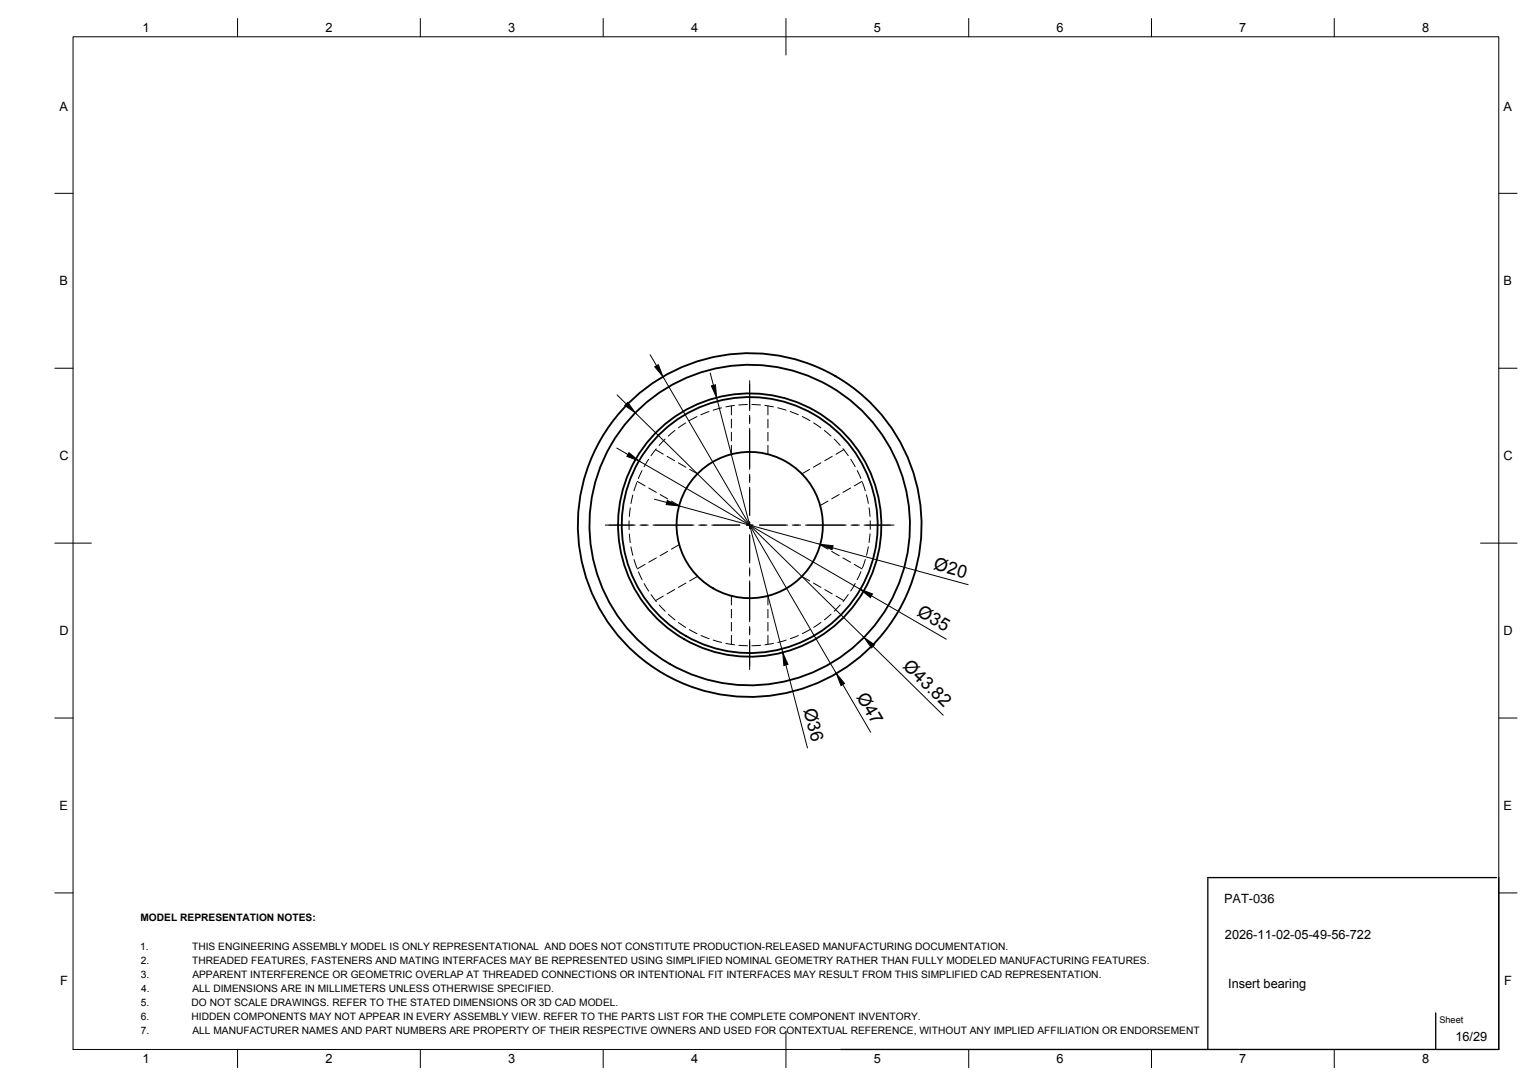
ISO-10303-21;
HEADER;
/* Generated by software containing ST-Developer
 * from STEP Tools, Inc. (www.steptools.com) 
 */

FILE_DESCRIPTION(
/* description */ ('Flange-mounted spindle'),
/* implementation_level */ '2;1');

FILE_NAME(
/* name */ 'Insert bearing.step',
/* time_stamp */ '2026-10-27T10:49:51-07:00',
/* author */ (''),
/* organization */ (''),
/* preprocessor_version */ 'ST-DEVELOPER v20.2',
/* originating_system */ 'Autodesk Translation Framework v15.17.0.0',
/* authorisation */ '');

FILE_SCHEMA (('AUTOMOTIVE_DESIGN { 1 0 10303 214 3 1 1 }'));
ENDSEC;

DATA;
#10=MECHANICAL_DESIGN_GEOMETRIC_PRESENTATION_REPRESENTATION('',(#348,#349),#11764);
#211=B_SPLINE_CURVE_WITH_KNOTS('',3,(#9556,#9557,#9558,#9559,#9560,#9561,
#9562,#9563,#9564,#9565),.UNSPECIFIED.,.F.,.F.,(4,2,2,2,4),(1.13193471301885,
1.22626174930539,1.32058878559194,1.41491753480854,1.50924628402513),
 .UNSPECIFIED.);
#212=B_SPLINE_CURVE_WITH_KNOTS('',3,(#9567,#9568,#9569,#9570,#9571,#9572,
#9573,#9574,#9575,#9576,#9577,#9578,#9579,#9580,#9581,#9582,#9583,#9584),
 .UNSPECIFIED.,.F.,.F.,(4,2,2,2,2,2,2,2,4),(0.377311571006283,0.471638607292829,
0.565965643579376,0.66029439279597,0.754623142012565,0.84895189122916,0.943280640445754,
1.0376076767323,1.13193471301885),.UNSPECIFIED.);
#213=B_SPLINE_CURVE_WITH_KNOTS('',3,(#9585,#9586,#9587,#9588,#9589,#9590,
#9591,#9592,#9593,#9594),.UNSPECIFIED.,.F.,.F.,(4,2,2,2,4),(1.50924628402513,
1.60357503324173,1.69790378245832,1.79223081874487,1.88655785503141),
 .UNSPECIFIED.);
#214=B_SPLINE_CURVE_WITH_KNOTS('',3,(#9597,#9598,#9599,#9600,#9601,#9602,
#9603,#9604,#9605,#9606,#9607,#9608,#9609,#9610,#9611,#9612,#9613,#9614,
#9615,#9616,#9617,#9618,#9619,#9620,#9621,#9622,#9623,#9624,#9625,#9626,
#9627,#9628,#9629,#9630),.UNSPECIFIED.,.T.,.F.,(4,2,2,2,2,2,2,2,2,2,2,2,
2,2,2,2,4),(0.,0.0946120580087934,0.189224116017587,0.283822945575014,0.378421775132442,
0.47302060468987,0.567619434247297,0.662231492256091,0.756843550264884,
0.851455608273677,0.94606766628247,1.0406664958399,1.13526532539733,1.22986415495475,
1.32446298451218,1.41907504252097,1.51368710052977),.UNSPECIFIED.);
#215=B_SPLINE_CURVE_WITH_KNOTS('',3,(#9633,#9634,#9635,#9636,#9637,#9638,
#9639,#9640,#9641,#9642,#9643,#9644,#9645,#9646,#9647,#9648,#9649,#9650,
#9651,#9652,#9653,#9654,#9655,#9656,#9657,#9658,#9659,#9660,#9661,#9662,
#9663,#9664,#9665,#9666),.UNSPECIFIED.,.T.,.F.,(4,2,2,2,2,2,2,2,2,2,2,2,
2,2,2,2,4),(0.,0.0946120580087934,0.189224116017587,0.283822945575014,0.378421775132442,
0.47302060468987,0.567619434247297,0.66223149225609,0.756843550264884,0.851455608273677,
0.94606766628247,1.0406664958399,1.13526532539733,1.22986415495475,1.32446298451218,
1.41907504252097,1.51368710052977),.UNSPECIFIED.);
#216=B_SPLINE_CURVE_WITH_KNOTS('',3,(#9670,#9671,#9672,#9673,#9674,#9675,
#9676,#9677,#9678,#9679),.UNSPECIFIED.,.F.,.F.,(4,2,2,2,4),(1.13193471301885,
1.22626174930539,1.32058878559194,1.41491753480854,1.50924628402513),
 .UNSPECIFIED.);
#217=B_SPLINE_CURVE_WITH_KNOTS('',3,(#9681,#9682,#9683,#9684,#9685,#9686,
#9687,#9688,#9689,#9690,#9691,#9692,#9693,#9694,#9695,#9696,#9697,#9698),
 .UNSPECIFIED.,.F.,.F.,(4,2,2,2,2,2,2,2,4),(0.377311571006283,0.47163860729283,
0.565965643579376,0.660294392795971,0.754623142012565,0.84895189122916,
0.943280640445755,1.0376076767323,1.13193471301885),.UNSPECIFIED.);
#218=B_SPLINE_CURVE_WITH_KNOTS('',3,(#9699,#9700,#9701,#9702,#9703,#9704,
#9705,#9706,#9707,#9708),.UNSPECIFIED.,.F.,.F.,(4,2,2,2,4),(1.50924628402513,
1.60357503324173,1.69790378245832,1.79223081874487,1.88655785503141),
 .UNSPECIFIED.);
#219=B_SPLINE_CURVE_WITH_KNOTS('',3,(#9717,#9718,#9719,#9720,#9721,#9722,
#9723,#9724,#9725,#9726,#9727,#9728,#9729,#9730,#9731,#9732,#9733,#9734),
 .UNSPECIFIED.,.F.,.F.,(4,2,2,2,2,2,2,2,4),(0.377311571006282,0.471638607292829,
0.565965643579376,0.660294392795971,0.754623142012565,0.84895189122916,
0.943280640445754,1.0376076767323,1.13193471301885),.UNSPECIFIED.);
#220=B_SPLINE_CURVE_WITH_KNOTS('',3,(#9736,#9737,#9738,#9739,#9740,#9741,
#9742,#9743,#9744,#9745),.UNSPECIFIED.,.F.,.F.,(4,2,2,2,4),(1.13193471301885,
1.22626174930539,1.32058878559194,1.41491753480854,1.50924628402513),
 .UNSPECIFIED.);
#221=B_SPLINE_CURVE_WITH_KNOTS('',3,(#9746,#9747,#9748,#9749,#9750,#9751,
#9752,#9753,#9754,#9755),.UNSPECIFIED.,.F.,.F.,(4,2,2,2,4),(1.50924628402513,
1.60357503324172,1.69790378245832,1.79223081874487,1.88655785503141),
 .UNSPECIFIED.);
#222=B_SPLINE_CURVE_WITH_KNOTS('',3,(#9758,#9759,#9760,#9761,#9762,#9763,
#9764,#9765,#9766,#9767,#9768,#9769,#9770,#9771,#9772,#9773,#9774,#9775),
 .UNSPECIFIED.,.F.,.F.,(4,2,2,2,2,2,2,2,4),(0.377311571006283,0.47163860729283,
0.565965643579376,0.660294392795971,0.754623142012565,0.84895189122916,
0.943280640445754,1.0376076767323,1.13193471301885),.UNSPECIFIED.);
#223=B_SPLINE_CURVE_WITH_KNOTS('',3,(#9777,#9778,#9779,#9780,#9781,#9782,
#9783,#9784,#9785,#9786),.UNSPECIFIED.,.F.,.F.,(4,2,2,2,4),(1.13193471301885,
1.22626174930539,1.32058878559194,1.41491753480854,1.50924628402513),
 .UNSPECIFIED.);
#224=B_SPLINE_CURVE_WITH_KNOTS('',3,(#9787,#9788,#9789,#9790,#9791,#9792,
#9793,#9794,#9795,#9796),.UNSPECIFIED.,.F.,.F.,(4,2,2,2,4),(1.50924628402513,
1.60357503324173,1.69790378245832,1.79223081874487,1.88655785503141),
 .UNSPECIFIED.);
#225=B_SPLINE_CURVE_WITH_KNOTS('',3,(#9799,#9800,#9801,#9802,#9803,#9804,
#9805,#9806,#9807,#9808,#9809,#9810,#9811,#9812,#9813,#9814,#9815,#9816),
 .UNSPECIFIED.,.F.,.F.,(4,2,2,2,2,2,2,2,4),(0.377311571006282,0.471638607292829,
0.565965643579376,0.66029439279597,0.754623142012565,0.84895189122916,0.943280640445754,
1.0376076767323,1.13193471301885),.UNSPECIFIED.);
#226=B_SPLINE_CURVE_WITH_KNOTS('',3,(#9818,#9819,#9820,#9821,#9822,#9823,
#9824,#9825,#9826,#9827),.UNSPECIFIED.,.F.,.F.,(4,2,2,2,4),(1.13193471301885,
1.22626174930539,1.32058878559194,1.41491753480854,1.50924628402513),
 .UNSPECIFIED.);
#227=B_SPLINE_CURVE_WITH_KNOTS('',3,(#9828,#9829,#9830,#9831,#9832,#9833,
#9834,#9835,#9836,#9837),.UNSPECIFIED.,.F.,.F.,(4,2,2,2,4),(1.50924628402513,
1.60357503324172,1.69790378245832,1.79223081874487,1.88655785503141),
 .UNSPECIFIED.);
#228=B_SPLINE_CURVE_WITH_KNOTS('',3,(#9840,#9841,#9842,#9843,#9844,#9845,
#9846,#9847,#9848,#9849,#9850,#9851,#9852,#9853,#9854,#9855,#9856,#9857),
 .UNSPECIFIED.,.F.,.F.,(4,2,2,2,2,2,2,2,4),(0.377311571006283,0.471638607292829,
0.565965643579376,0.660294392795971,0.754623142012565,0.84895189122916,
0.943280640445755,1.0376076767323,1.13193471301885),.UNSPECIFIED.);
#229=B_SPLINE_CURVE_WITH_KNOTS('',3,(#9859,#9860,#9861,#9862,#9863,#9864,
#9865,#9866,#9867,#9868),.UNSPECIFIED.,.F.,.F.,(4,2,2,2,4),(1.13193471301885,
1.22626174930539,1.32058878559194,1.41491753480854,1.50924628402513),
 .UNSPECIFIED.);
#230=B_SPLINE_CURVE_WITH_KNOTS('',3,(#9869,#9870,#9871,#9872,#9873,#9874,
#9875,#9876,#9877,#9878),.UNSPECIFIED.,.F.,.F.,(4,2,2,2,4),(1.50924628402513,
1.60357503324172,1.69790378245832,1.79223081874487,1.88655785503141),
 .UNSPECIFIED.);
#231=B_SPLINE_CURVE_WITH_KNOTS('',3,(#9882,#9883,#9884,#9885,#9886,#9887,
#9888,#9889,#9890,#9891,#9892,#9893,#9894,#9895,#9896,#9897,#9898,#9899,
#9900,#9901,#9902,#9903,#9904,#9905,#9906,#9907,#9908,#9909,#9910,#9911,
#9912,#9913,#9914,#9915),.UNSPECIFIED.,.T.,.F.,(4,2,2,2,2,2,2,2,2,2,2,2,
2,2,2,2,4),(0.,0.0946120580087934,0.189224116017587,0.283822945575014,0.378421775132442,
0.47302060468987,0.567619434247297,0.66223149225609,0.756843550264884,0.851455608273677,
0.94606766628247,1.0406664958399,1.13526532539733,1.22986415495475,1.32446298451218,
1.41907504252097,1.51368710052977),.UNSPECIFIED.);
#232=B_SPLINE_CURVE_WITH_KNOTS('',3,(#9918,#9919,#9920,#9921,#9922,#9923,
#9924,#9925,#9926,#9927,#9928,#9929,#9930,#9931,#9932,#9933,#9934,#9935,
#9936,#9937,#9938,#9939,#9940,#9941,#9942,#9943,#9944,#9945,#9946,#9947,
#9948,#9949,#9950,#9951),.UNSPECIFIED.,.T.,.F.,(4,2,2,2,2,2,2,2,2,2,2,2,
2,2,2,2,4),(0.,0.0946120580087934,0.189224116017587,0.283822945575014,0.378421775132442,
0.47302060468987,0.567619434247297,0.66223149225609,0.756843550264884,0.851455608273677,
0.94606766628247,1.0406664958399,1.13526532539733,1.22986415495475,1.32446298451218,
1.41907504252097,1.51368710052977),.UNSPECIFIED.);
#233=B_SPLINE_CURVE_WITH_KNOTS('',3,(#9956,#9957,#9958,#9959,#9960,#9961,
#9962,#9963,#9964,#9965,#9966,#9967,#9968,#9969,#9970,#9971,#9972,#9973,
#9974,#9975,#9976,#9977,#9978,#9979,#9980,#9981,#9982,#9983,#9984,#9985,
#9986,#9987,#9988,#9989),.UNSPECIFIED.,.T.,.F.,(4,2,2,2,2,2,2,2,2,2,2,2,
2,2,2,2,4),(0.,0.0946120580087934,0.189224116017587,0.283822945575014,0.378421775132442,
0.47302060468987,0.567619434247297,0.66223149225609,0.756843550264884,0.851455608273677,
0.94606766628247,1.0406664958399,1.13526532539733,1.22986415495475,1.32446298451218,
1.41907504252097,1.51368710052977),.UNSPECIFIED.);
#234=B_SPLINE_CURVE_WITH_KNOTS('',3,(#9992,#9993,#9994,#9995,#9996,#9997,
#9998,#9999,#10000,#10001,#10002,#10003,#10004,#10005,#10006,#10007,#10008,
#10009,#10010,#10011,#10012,#10013,#10014,#10015,#10016,#10017,#10018,#10019,
#10020,#10021,#10022,#10023,#10024,#10025),.UNSPECIFIED.,.T.,.F.,(4,2,2,
2,2,2,2,2,2,2,2,2,2,2,2,2,4),(0.,0.0946120580087934,0.189224116017587,0.283822945575014,
0.378421775132442,0.47302060468987,0.567619434247297,0.66223149225609,0.756843550264884,
0.851455608273677,0.94606766628247,1.0406664958399,1.13526532539733,1.22986415495475,
1.32446298451218,1.41907504252097,1.51368710052977),.UNSPECIFIED.);
#262=SPHERICAL_SURFACE('',#6624,2.35);
#294=SHAPE_REPRESENTATION_RELATIONSHIP('SRR','None',#11891,#321);
#321=ADVANCED_BREP_SHAPE_REPRESENTATION('',(#375,#376),#11746);
#348=STYLED_ITEM('',(#12099),#375);
#349=STYLED_ITEM('',(#12099),#376);
#375=MANIFOLD_SOLID_BREP('Body1',#6141);
#376=MANIFOLD_SOLID_BREP('Body2',#6142);
#432=FACE_BOUND('',#1150,.T.);
#433=FACE_BOUND('',#1152,.T.);
#434=FACE_BOUND('',#1153,.T.);
#435=FACE_BOUND('',#1155,.T.);
#436=FACE_BOUND('',#1159,.T.);
#437=FACE_BOUND('',#1160,.T.);
#438=FACE_BOUND('',#1161,.T.);
#439=FACE_BOUND('',#1162,.T.);
#440=FACE_BOUND('',#1163,.T.);
#441=FACE_BOUND('',#1164,.T.);
#442=FACE_BOUND('',#1170,.T.);
#443=FACE_BOUND('',#1172,.T.);
#444=FACE_BOUND('',#1175,.T.);
#445=FACE_BOUND('',#1177,.T.);
#446=FACE_BOUND('',#1178,.T.);
#447=FACE_BOUND('',#1179,.T.);
#448=FACE_BOUND('',#1180,.T.);
#449=FACE_BOUND('',#1181,.T.);
#450=FACE_BOUND('',#1182,.T.);
#563=PLANE('',#6622);
#564=PLANE('',#6627);
#565=PLANE('',#6637);
#566=PLANE('',#6639);
#567=PLANE('',#6643);
#762=FACE_OUTER_BOUND('',#1148,.T.);
#763=FACE_OUTER_BOUND('',#1149,.T.);
#764=FACE_OUTER_BOUND('',#1151,.T.);
#765=FACE_OUTER_BOUND('',#1154,.T.);
#766=FACE_OUTER_BOUND('',#1156,.T.);
#767=FACE_OUTER_BOUND('',#1157,.T.);
#768=FACE_OUTER_BOUND('',#1158,.T.);
#769=FACE_OUTER_BOUND('',#1165,.T.);
#770=FACE_OUTER_BOUND('',#1166,.T.);
#771=FACE_OUTER_BOUND('',#1167,.T.);
#772=FACE_OUTER_BOUND('',#1168,.T.);
#773=FACE_OUTER_BOUND('',#1169,.T.);
#774=FACE_OUTER_BOUND('',#1171,.T.);
#775=FACE_OUTER_BOUND('',#1173,.T.);
#776=FACE_OUTER_BOUND('',#1174,.T.);
#777=FACE_OUTER_BOUND('',#1176,.T.);
#1148=EDGE_LOOP('',(#4373,#4374,#4375,#4376));
#1149=EDGE_LOOP('',(#4377));
#1150=EDGE_LOOP('',(#4378));
#1151=EDGE_LOOP('',(#4379,#4380));
#1152=EDGE_LOOP('',(#4381));
#1153=EDGE_LOOP('',(#4382));
#1154=EDGE_LOOP('',(#4383));
#1155=EDGE_LOOP('',(#4384));
#1156=EDGE_LOOP('',(#4385,#4386,#4387,#4388,#4389,#4390));
#1157=EDGE_LOOP('',(#4391,#4392,#4393,#4394,#4395,#4396));
#1158=EDGE_LOOP('',(#4397,#4398,#4399,#4400));
#1159=EDGE_LOOP('',(#4401,#4402,#4403));
#1160=EDGE_LOOP('',(#4404,#4405,#4406));
#1161=EDGE_LOOP('',(#4407,#4408,#4409));
#1162=EDGE_LOOP('',(#4410,#4411,#4412));
#1163=EDGE_LOOP('',(#4413,#4414,#4415));
#1164=EDGE_LOOP('',(#4416,#4417,#4418));
#1165=EDGE_LOOP('',(#4419,#4420,#4421,#4422,#4423,#4424));
#1166=EDGE_LOOP('',(#4425,#4426,#4427,#4428,#4429,#4430));
#1167=EDGE_LOOP('',(#4431,#4432,#4433,#4434,#4435,#4436));
#1168=EDGE_LOOP('',(#4437,#4438,#4439,#4440,#4441,#4442));
#1169=EDGE_LOOP('',(#4443));
#1170=EDGE_LOOP('',(#4444));
#1171=EDGE_LOOP('',(#4445));
#1172=EDGE_LOOP('',(#4446));
#1173=EDGE_LOOP('',(#4447,#4448,#4449,#4450));
#1174=EDGE_LOOP('',(#4451));
#1175=EDGE_LOOP('',(#4452));
#1176=EDGE_LOOP('',(#4453,#4454,#4455,#4456));
#1177=EDGE_LOOP('',(#4457));
#1178=EDGE_LOOP('',(#4458));
#1179=EDGE_LOOP('',(#4459));
#1180=EDGE_LOOP('',(#4460));
#1181=EDGE_LOOP('',(#4461));
#1182=EDGE_LOOP('',(#4462));
#1605=LINE('',#9541,#2027);
#1606=LINE('',#9596,#2028);
#1607=LINE('',#9668,#2029);
#1608=LINE('',#9713,#2030);
#1609=LINE('',#9881,#2031);
#1610=LINE('',#9952,#2032);
#1611=LINE('',#9955,#2033);
#1612=LINE('',#10026,#2034);
#1613=LINE('',#10036,#2035);
#1614=LINE('',#10041,#2036);
#2027=VECTOR('',#7658,1.8);
#2028=VECTOR('',#7675,0.25);
#2029=VECTOR('',#7678,0.25);
#2030=VECTOR('',#7683,1.65);
#2031=VECTOR('',#7688,0.25);
#2032=VECTOR('',#7691,0.25);
#2033=VECTOR('',#7694,0.25);
#2034=VECTOR('',#7697,0.25);
#2035=VECTOR('',#7710,1.75);
#2036=VECTOR('',#7717,1.);
#2381=CIRCLE('',#6620,1.8);
#2382=CIRCLE('',#6621,1.8);
#2383=CIRCLE('',#6623,2.19089023002066);
#2384=CIRCLE('',#6625,2.35);
#2385=CIRCLE('',#6626,2.19089023002066);
#2386=CIRCLE('',#6631,1.65);
#2387=CIRCLE('',#6632,1.65);
#2388=CIRCLE('',#6638,1.);
#2389=CIRCLE('',#6640,1.75);
#2390=CIRCLE('',#6642,1.75);
#2391=CIRCLE('',#6644,1.);
#2772=VERTEX_POINT('',#9538);
#2773=VERTEX_POINT('',#9540);
#2774=VERTEX_POINT('',#9544);
#2775=VERTEX_POINT('',#9547);
#2776=VERTEX_POINT('',#9548);
#2777=VERTEX_POINT('',#9550);
#2778=VERTEX_POINT('',#9554);
#2779=VERTEX_POINT('',#9555);
#2780=VERTEX_POINT('',#9566);
#2781=VERTEX_POINT('',#9595);
#2782=VERTEX_POINT('',#9632);
#2783=VERTEX_POINT('',#9667);
#2784=VERTEX_POINT('',#9669);
#2785=VERTEX_POINT('',#9680);
#2786=VERTEX_POINT('',#9710);
#2787=VERTEX_POINT('',#9712);
#2788=VERTEX_POINT('',#9715);
#2789=VERTEX_POINT('',#9716);
#2790=VERTEX_POINT('',#9735);
#2791=VERTEX_POINT('',#9756);
#2792=VERTEX_POINT('',#9757);
#2793=VERTEX_POINT('',#9776);
#2794=VERTEX_POINT('',#9797);
#2795=VERTEX_POINT('',#9798);
#2796=VERTEX_POINT('',#9817);
#2797=VERTEX_POINT('',#9838);
#2798=VERTEX_POINT('',#9839);
#2799=VERTEX_POINT('',#9858);
#2800=VERTEX_POINT('',#9880);
#2801=VERTEX_POINT('',#9917);
#2802=VERTEX_POINT('',#9954);
#2803=VERTEX_POINT('',#9991);
#2804=VERTEX_POINT('',#10028);
#2805=VERTEX_POINT('',#10031);
#2806=VERTEX_POINT('',#10034);
#2807=VERTEX_POINT('',#10038);
#3379=EDGE_CURVE('',#2772,#2772,#2381,.T.);
#3380=EDGE_CURVE('',#2772,#2773,#1605,.T.);
#3381=EDGE_CURVE('',#2773,#2773,#2382,.T.);
#3382=EDGE_CURVE('',#2774,#2774,#2383,.T.);
#3383=EDGE_CURVE('',#2775,#2776,#2384,.T.);
#3384=EDGE_CURVE('',#2777,#2777,#2385,.T.);
#3385=EDGE_CURVE('',#2778,#2779,#211,.T.);
#3386=EDGE_CURVE('',#2780,#2778,#212,.T.);
#3387=EDGE_CURVE('',#2779,#2780,#213,.T.);
#3388=EDGE_CURVE('',#2779,#2781,#1606,.T.);
#3389=EDGE_CURVE('',#2781,#2781,#214,.T.);
#3390=EDGE_CURVE('',#2782,#2782,#215,.T.);
#3391=EDGE_CURVE('',#2782,#2783,#1607,.T.);
#3392=EDGE_CURVE('',#2784,#2783,#216,.T.);
#3393=EDGE_CURVE('',#2785,#2784,#217,.T.);
#3394=EDGE_CURVE('',#2783,#2785,#218,.T.);
#3395=EDGE_CURVE('',#2786,#2786,#2386,.T.);
#3396=EDGE_CURVE('',#2786,#2787,#1608,.T.);
#3397=EDGE_CURVE('',#2787,#2787,#2387,.T.);
#3398=EDGE_CURVE('',#2788,#2789,#219,.T.);
#3399=EDGE_CURVE('',#2789,#2790,#220,.T.);
#3400=EDGE_CURVE('',#2790,#2788,#221,.T.);
#3401=EDGE_CURVE('',#2791,#2792,#222,.T.);
#3402=EDGE_CURVE('',#2792,#2793,#223,.T.);
#3403=EDGE_CURVE('',#2793,#2791,#224,.T.);
#3404=EDGE_CURVE('',#2794,#2795,#225,.T.);
#3405=EDGE_CURVE('',#2795,#2796,#226,.T.);
#3406=EDGE_CURVE('',#2796,#2794,#227,.T.);
#3407=EDGE_CURVE('',#2797,#2798,#228,.T.);
#3408=EDGE_CURVE('',#2798,#2799,#229,.T.);
#3409=EDGE_CURVE('',#2799,#2797,#230,.T.);
#3410=EDGE_CURVE('',#2790,#2800,#1609,.T.);
#3411=EDGE_CURVE('',#2800,#2800,#231,.T.);
#3412=EDGE_CURVE('',#2801,#2801,#232,.T.);
#3413=EDGE_CURVE('',#2801,#2793,#1610,.T.);
#3414=EDGE_CURVE('',#2796,#2802,#1611,.T.);
#3415=EDGE_CURVE('',#2802,#2802,#233,.T.);
#3416=EDGE_CURVE('',#2803,#2803,#234,.T.);
#3417=EDGE_CURVE('',#2803,#2799,#1612,.T.);
#3418=EDGE_CURVE('',#2804,#2804,#2388,.T.);
#3419=EDGE_CURVE('',#2805,#2805,#2389,.T.);
#3420=EDGE_CURVE('',#2806,#2806,#2390,.T.);
#3421=EDGE_CURVE('',#2806,#2805,#1613,.T.);
#3422=EDGE_CURVE('',#2807,#2807,#2391,.T.);
#3423=EDGE_CURVE('',#2807,#2804,#1614,.T.);
#4373=ORIENTED_EDGE('',*,*,#3379,.T.);
#4374=ORIENTED_EDGE('',*,*,#3380,.T.);
#4375=ORIENTED_EDGE('',*,*,#3381,.F.);
#4376=ORIENTED_EDGE('',*,*,#3380,.F.);
#4377=ORIENTED_EDGE('',*,*,#3382,.F.);
#4378=ORIENTED_EDGE('',*,*,#3381,.T.);
#4379=ORIENTED_EDGE('',*,*,#3383,.T.);
#4380=ORIENTED_EDGE('',*,*,#3383,.F.);
#4381=ORIENTED_EDGE('',*,*,#3382,.T.);
#4382=ORIENTED_EDGE('',*,*,#3384,.F.);
#4383=ORIENTED_EDGE('',*,*,#3384,.T.);
#4384=ORIENTED_EDGE('',*,*,#3379,.F.);
#4385=ORIENTED_EDGE('',*,*,#3385,.F.);
#4386=ORIENTED_EDGE('',*,*,#3386,.F.);
#4387=ORIENTED_EDGE('',*,*,#3387,.F.);
#4388=ORIENTED_EDGE('',*,*,#3388,.T.);
#4389=ORIENTED_EDGE('',*,*,#3389,.F.);
#4390=ORIENTED_EDGE('',*,*,#3388,.F.);
#4391=ORIENTED_EDGE('',*,*,#3390,.F.);
#4392=ORIENTED_EDGE('',*,*,#3391,.T.);
#4393=ORIENTED_EDGE('',*,*,#3392,.F.);
#4394=ORIENTED_EDGE('',*,*,#3393,.F.);
#4395=ORIENTED_EDGE('',*,*,#3394,.F.);
#4396=ORIENTED_EDGE('',*,*,#3391,.F.);
#4397=ORIENTED_EDGE('',*,*,#3395,.F.);
#4398=ORIENTED_EDGE('',*,*,#3396,.T.);
#4399=ORIENTED_EDGE('',*,*,#3397,.T.);
#4400=ORIENTED_EDGE('',*,*,#3396,.F.);
#4401=ORIENTED_EDGE('',*,*,#3386,.T.);
#4402=ORIENTED_EDGE('',*,*,#3385,.T.);
#4403=ORIENTED_EDGE('',*,*,#3387,.T.);
#4404=ORIENTED_EDGE('',*,*,#3393,.T.);
#4405=ORIENTED_EDGE('',*,*,#3392,.T.);
#4406=ORIENTED_EDGE('',*,*,#3394,.T.);
#4407=ORIENTED_EDGE('',*,*,#3398,.T.);
#4408=ORIENTED_EDGE('',*,*,#3399,.T.);
#4409=ORIENTED_EDGE('',*,*,#3400,.T.);
#4410=ORIENTED_EDGE('',*,*,#3401,.T.);
#4411=ORIENTED_EDGE('',*,*,#3402,.T.);
#4412=ORIENTED_EDGE('',*,*,#3403,.T.);
#4413=ORIENTED_EDGE('',*,*,#3404,.T.);
#4414=ORIENTED_EDGE('',*,*,#3405,.T.);
#4415=ORIENTED_EDGE('',*,*,#3406,.T.);
#4416=ORIENTED_EDGE('',*,*,#3407,.T.);
#4417=ORIENTED_EDGE('',*,*,#3408,.T.);
#4418=ORIENTED_EDGE('',*,*,#3409,.T.);
#4419=ORIENTED_EDGE('',*,*,#3399,.F.);
#4420=ORIENTED_EDGE('',*,*,#3398,.F.);
#4421=ORIENTED_EDGE('',*,*,#3400,.F.);
#4422=ORIENTED_EDGE('',*,*,#3410,.T.);
#4423=ORIENTED_EDGE('',*,*,#3411,.F.);
#4424=ORIENTED_EDGE('',*,*,#3410,.F.);
#4425=ORIENTED_EDGE('',*,*,#3412,.F.);
#4426=ORIENTED_EDGE('',*,*,#3413,.T.);
#4427=ORIENTED_EDGE('',*,*,#3402,.F.);
#4428=ORIENTED_EDGE('',*,*,#3401,.F.);
#4429=ORIENTED_EDGE('',*,*,#3403,.F.);
#4430=ORIENTED_EDGE('',*,*,#3413,.F.);
#4431=ORIENTED_EDGE('',*,*,#3405,.F.);
#4432=ORIENTED_EDGE('',*,*,#3404,.F.);
#4433=ORIENTED_EDGE('',*,*,#3406,.F.);
#4434=ORIENTED_EDGE('',*,*,#3414,.T.);
#4435=ORIENTED_EDGE('',*,*,#3415,.F.);
#4436=ORIENTED_EDGE('',*,*,#3414,.F.);
#4437=ORIENTED_EDGE('',*,*,#3416,.F.);
#4438=ORIENTED_EDGE('',*,*,#3417,.T.);
#4439=ORIENTED_EDGE('',*,*,#3408,.F.);
#4440=ORIENTED_EDGE('',*,*,#3407,.F.);
#4441=ORIENTED_EDGE('',*,*,#3409,.F.);
#4442=ORIENTED_EDGE('',*,*,#3417,.F.);
#4443=ORIENTED_EDGE('',*,*,#3397,.F.);
#4444=ORIENTED_EDGE('',*,*,#3418,.T.);
#4445=ORIENTED_EDGE('',*,*,#3419,.F.);
#4446=ORIENTED_EDGE('',*,*,#3395,.T.);
#4447=ORIENTED_EDGE('',*,*,#3420,.F.);
#4448=ORIENTED_EDGE('',*,*,#3421,.T.);
#4449=ORIENTED_EDGE('',*,*,#3419,.T.);
#4450=ORIENTED_EDGE('',*,*,#3421,.F.);
#4451=ORIENTED_EDGE('',*,*,#3420,.T.);
#4452=ORIENTED_EDGE('',*,*,#3422,.F.);
#4453=ORIENTED_EDGE('',*,*,#3422,.T.);
#4454=ORIENTED_EDGE('',*,*,#3423,.T.);
#4455=ORIENTED_EDGE('',*,*,#3418,.F.);
#4456=ORIENTED_EDGE('',*,*,#3423,.F.);
#4457=ORIENTED_EDGE('',*,*,#3390,.T.);
#4458=ORIENTED_EDGE('',*,*,#3389,.T.);
#4459=ORIENTED_EDGE('',*,*,#3412,.T.);
#4460=ORIENTED_EDGE('',*,*,#3411,.T.);
#4461=ORIENTED_EDGE('',*,*,#3416,.T.);
#4462=ORIENTED_EDGE('',*,*,#3415,.T.);
#5652=CYLINDRICAL_SURFACE('',#6619,1.8);
#5653=CYLINDRICAL_SURFACE('',#6628,0.25);
#5654=CYLINDRICAL_SURFACE('',#6629,0.25);
#5655=CYLINDRICAL_SURFACE('',#6630,1.65);
#5656=CYLINDRICAL_SURFACE('',#6633,0.25);
#5657=CYLINDRICAL_SURFACE('',#6634,0.25);
#5658=CYLINDRICAL_SURFACE('',#6635,0.25);
#5659=CYLINDRICAL_SURFACE('',#6636,0.25);
#5660=CYLINDRICAL_SURFACE('',#6641,1.75);
#5661=CYLINDRICAL_SURFACE('',#6645,1.);
#5873=ADVANCED_FACE('',(#762),#5652,.F.);
#5874=ADVANCED_FACE('',(#763,#432),#563,.T.);
#5875=ADVANCED_FACE('',(#764,#433,#434),#262,.T.);
#5876=ADVANCED_FACE('',(#765,#435),#564,.T.);
#5877=ADVANCED_FACE('',(#766),#5653,.F.);
#5878=ADVANCED_FACE('',(#767),#5654,.F.);
#5879=ADVANCED_FACE('',(#768,#436,#437,#438,#439,#440,#441),#5655,.T.);
#5880=ADVANCED_FACE('',(#769),#5656,.F.);
#5881=ADVANCED_FACE('',(#770),#5657,.F.);
#5882=ADVANCED_FACE('',(#771),#5658,.F.);
#5883=ADVANCED_FACE('',(#772),#5659,.F.);
#5884=ADVANCED_FACE('',(#773,#442),#565,.T.);
#5885=ADVANCED_FACE('',(#774,#443),#566,.T.);
#5886=ADVANCED_FACE('',(#775),#5660,.T.);
#5887=ADVANCED_FACE('',(#776,#444),#567,.T.);
#5888=ADVANCED_FACE('',(#777,#445,#446,#447,#448,#449,#450),#5661,.F.);
#6141=CLOSED_SHELL('',(#5873,#5874,#5875,#5876));
#6142=CLOSED_SHELL('',(#5877,#5878,#5879,#5880,#5881,#5882,#5883,#5884,
#5885,#5886,#5887,#5888));
#6618=AXIS2_PLACEMENT_3D('',#9536,#7652,#7653);
#6619=AXIS2_PLACEMENT_3D('',#9537,#7654,#7655);
#6620=AXIS2_PLACEMENT_3D('',#9539,#7656,#7657);
#6621=AXIS2_PLACEMENT_3D('',#9542,#7659,#7660);
#6622=AXIS2_PLACEMENT_3D('',#9543,#7661,#7662);
#6623=AXIS2_PLACEMENT_3D('',#9545,#7663,#7664);
#6624=AXIS2_PLACEMENT_3D('',#9546,#7665,#7666);
#6625=AXIS2_PLACEMENT_3D('',#9549,#7667,#7668);
#6626=AXIS2_PLACEMENT_3D('',#9551,#7669,#7670);
#6627=AXIS2_PLACEMENT_3D('',#9552,#7671,#7672);
#6628=AXIS2_PLACEMENT_3D('',#9553,#7673,#7674);
#6629=AXIS2_PLACEMENT_3D('',#9631,#7676,#7677);
#6630=AXIS2_PLACEMENT_3D('',#9709,#7679,#7680);
#6631=AXIS2_PLACEMENT_3D('',#9711,#7681,#7682);
#6632=AXIS2_PLACEMENT_3D('',#9714,#7684,#7685);
#6633=AXIS2_PLACEMENT_3D('',#9879,#7686,#7687);
#6634=AXIS2_PLACEMENT_3D('',#9916,#7689,#7690);
#6635=AXIS2_PLACEMENT_3D('',#9953,#7692,#7693);
#6636=AXIS2_PLACEMENT_3D('',#9990,#7695,#7696);
#6637=AXIS2_PLACEMENT_3D('',#10027,#7698,#7699);
#6638=AXIS2_PLACEMENT_3D('',#10029,#7700,#7701);
#6639=AXIS2_PLACEMENT_3D('',#10030,#7702,#7703);
#6640=AXIS2_PLACEMENT_3D('',#10032,#7704,#7705);
#6641=AXIS2_PLACEMENT_3D('',#10033,#7706,#7707);
#6642=AXIS2_PLACEMENT_3D('',#10035,#7708,#7709);
#6643=AXIS2_PLACEMENT_3D('',#10037,#7711,#7712);
#6644=AXIS2_PLACEMENT_3D('',#10039,#7713,#7714);
#6645=AXIS2_PLACEMENT_3D('',#10040,#7715,#7716);
#7652=DIRECTION('axis',(0.,0.,1.));
#7653=DIRECTION('refdir',(1.,0.,0.));
#7654=DIRECTION('center_axis',(0.,-1.,0.));
#7655=DIRECTION('ref_axis',(1.,0.,0.));
#7656=DIRECTION('center_axis',(0.,-1.,0.));
#7657=DIRECTION('ref_axis',(1.,0.,0.));
#7658=DIRECTION('',(0.,1.,0.));
#7659=DIRECTION('center_axis',(0.,-1.,0.));
#7660=DIRECTION('ref_axis',(1.,0.,0.));
#7661=DIRECTION('center_axis',(0.,1.,0.));
#7662=DIRECTION('ref_axis',(0.,0.,1.));
#7663=DIRECTION('center_axis',(0.,-1.,0.));
#7664=DIRECTION('ref_axis',(1.,0.,0.));
#7665=DIRECTION('center_axis',(6.12323399573677E-17,0.,1.));
#7666=DIRECTION('ref_axis',(1.,0.,0.));
#7667=DIRECTION('center_axis',(1.22464679914735E-16,-1.,0.));
#7668=DIRECTION('ref_axis',(-1.,-1.22464679914735E-16,0.));
#7669=DIRECTION('center_axis',(0.,-1.,0.));
#7670=DIRECTION('ref_axis',(1.,0.,0.));
#7671=DIRECTION('center_axis',(0.,-1.,0.));
#7672=DIRECTION('ref_axis',(0.,0.,-1.));
#7673=DIRECTION('center_axis',(-0.866025403784438,0.,-0.5));
#7674=DIRECTION('ref_axis',(-0.5,0.,0.866025403784438));
#7675=DIRECTION('',(-0.866025403784438,0.,-0.5));
#7676=DIRECTION('center_axis',(-0.866025403784438,0.,-0.5));
#7677=DIRECTION('ref_axis',(-0.5,0.,0.866025403784438));
#7678=DIRECTION('',(-0.866025403784438,0.,-0.5));
#7679=DIRECTION('center_axis',(0.,-1.,0.));
#7680=DIRECTION('ref_axis',(1.,0.,0.));
#7681=DIRECTION('center_axis',(0.,-1.,0.));
#7682=DIRECTION('ref_axis',(1.,0.,0.));
#7683=DIRECTION('',(0.,1.,0.));
#7684=DIRECTION('center_axis',(0.,-1.,0.));
#7685=DIRECTION('ref_axis',(1.,0.,0.));
#7686=DIRECTION('center_axis',(0.866025403784439,0.,-0.5));
#7687=DIRECTION('ref_axis',(-0.5,0.,-0.866025403784439));
#7688=DIRECTION('',(0.866025403784439,0.,-0.5));
#7689=DIRECTION('center_axis',(0.866025403784439,0.,-0.5));
#7690=DIRECTION('ref_axis',(-0.5,0.,-0.866025403784439));
#7691=DIRECTION('',(0.866025403784439,0.,-0.5));
#7692=DIRECTION('center_axis',(0.,0.,1.));
#7693=DIRECTION('ref_axis',(1.,0.,0.));
#7694=DIRECTION('',(0.,0.,1.));
#7695=DIRECTION('center_axis',(0.,0.,1.));
#7696=DIRECTION('ref_axis',(1.,0.,0.));
#7697=DIRECTION('',(0.,0.,1.));
#7698=DIRECTION('center_axis',(0.,1.,0.));
#7699=DIRECTION('ref_axis',(0.,0.,1.));
#7700=DIRECTION('center_axis',(0.,-1.,0.));
#7701=DIRECTION('ref_axis',(1.,0.,0.));
#7702=DIRECTION('center_axis',(0.,1.,0.));
#7703=DIRECTION('ref_axis',(0.,0.,1.));
#7704=DIRECTION('center_axis',(0.,-1.,0.));
#7705=DIRECTION('ref_axis',(1.,0.,0.));
#7706=DIRECTION('center_axis',(0.,-1.,0.));
#7707=DIRECTION('ref_axis',(1.,0.,0.));
#7708=DIRECTION('center_axis',(0.,-1.,0.));
#7709=DIRECTION('ref_axis',(1.,0.,0.));
#7710=DIRECTION('',(0.,1.,0.));
#7711=DIRECTION('center_axis',(0.,-1.,0.));
#7712=DIRECTION('ref_axis',(0.,0.,-1.));
#7713=DIRECTION('center_axis',(0.,-1.,0.));
#7714=DIRECTION('ref_axis',(1.,0.,0.));
#7715=DIRECTION('center_axis',(0.,-1.,0.));
#7716=DIRECTION('ref_axis',(1.,0.,0.));
#7717=DIRECTION('',(0.,1.,0.));
#9536=CARTESIAN_POINT('',(0.,0.,0.));
#9537=CARTESIAN_POINT('Origin',(0.,0.,0.));
#9538=CARTESIAN_POINT('',(-1.8,-0.85,-2.20436423846524E-16));
#9539=CARTESIAN_POINT('Origin',(0.,-0.85,0.));
#9540=CARTESIAN_POINT('',(-1.8,0.85,-2.20436423846524E-16));
#9541=CARTESIAN_POINT('',(-1.8,0.,-2.20436423846524E-16));
#9542=CARTESIAN_POINT('Origin',(0.,0.85,0.));
#9543=CARTESIAN_POINT('Origin',(2.19089023002066,0.85,0.));
#9544=CARTESIAN_POINT('',(2.19089023002066,0.85,0.));
#9545=CARTESIAN_POINT('Origin',(0.,0.85,0.));
#9546=CARTESIAN_POINT('Origin',(3.99680288865056E-15,0.,0.));
#9547=CARTESIAN_POINT('',(3.85290688975075E-15,-1.76221774462768E-32,2.35));
#9548=CARTESIAN_POINT('',(3.85290688975075E-15,-1.76221774462768E-32,-2.35));
#9549=CARTESIAN_POINT('Origin',(3.99680288865056E-15,0.,0.));
#9550=CARTESIAN_POINT('',(2.19089023002066,-0.85,0.));
#9551=CARTESIAN_POINT('Origin',(0.,-0.85,0.));
#9552=CARTESIAN_POINT('Origin',(1.8,-0.85,0.));
#9553=CARTESIAN_POINT('Origin',(0.,1.55,0.));
#9554=CARTESIAN_POINT('',(1.42894191624432,1.8,0.825000000000001));
#9555=CARTESIAN_POINT('',(1.53744468918255,1.55,0.598968970568896));
#9556=CARTESIAN_POINT('Ctrl Pts',(1.42894191624432,1.8,0.825000000000001));
#9557=CARTESIAN_POINT('Ctrl Pts',(1.44466308895875,1.8,0.797770130104052));
#9558=CARTESIAN_POINT('Ctrl Pts',(1.46055812562105,1.79370633789704,0.768258557763732));
#9559=CARTESIAN_POINT('Ctrl Pts',(1.48824888379079,1.76817777258318,0.713138492740816));
#9560=CARTESIAN_POINT('Ctrl Pts',(1.50008999307766,1.74894552961493,0.687551581002689));
#9561=CARTESIAN_POINT('Ctrl Pts',(1.51812136280714,1.70460745840382,0.646764802471699));
#9562=CARTESIAN_POINT('Ctrl Pts',(1.52552758004446,1.67652816181843,0.628833667319578));
#9563=CARTESIAN_POINT('Ctrl Pts',(1.53516661651472,1.61494799959182,0.604921184808251));
#9564=CARTESIAN_POINT('Ctrl Pts',(1.53744468918255,1.58144291640553,0.598968970568896));
#9565=CARTESIAN_POINT('Ctrl Pts',(1.53744468918255,1.55,0.598968970568896));
#9566=CARTESIAN_POINT('',(1.42894191624432,1.3,0.825000000000001));
#9567=CARTESIAN_POINT('Ctrl Pts',(1.42894191624432,1.3,0.825000000000001));
#9568=CARTESIAN_POINT('Ctrl Pts',(1.4132207435299,1.3,0.852229869895949));
#9569=CARTESIAN_POINT('Ctrl Pts',(1.39561049050871,1.30629366210296,0.880751161609749));
#9570=CARTESIAN_POINT('Ctrl Pts',(1.36172049302549,1.33182222741682,0.932292094146256));
#9571=CARTESIAN_POINT('Ctrl Pts',(1.34548213209931,1.35105447038507,0.955340251466734));
#9572=CARTESIAN_POINT('Ctrl Pts',(1.31917543061769,1.39539254159618,0.99134926498299));
#9573=CARTESIAN_POINT('Ctrl Pts',(1.30734972067592,1.42347183818157,1.00672880483252));
#9574=CARTESIAN_POINT('Ctrl Pts',(1.29146042158868,1.48505200040818,1.02703269653942));
#9575=CARTESIAN_POINT('Ctrl Pts',(1.28744468918255,1.51855708359447,1.03198167246111));
#9576=CARTESIAN_POINT('Ctrl Pts',(1.28744468918255,1.58144291640553,1.03198167246111));
#9577=CARTESIAN_POINT('Ctrl Pts',(1.29146042158868,1.61494799959182,1.02703269653942));
#9578=CARTESIAN_POINT('Ctrl Pts',(1.30734972067592,1.67652816181843,1.00672880483252));
#9579=CARTESIAN_POINT('Ctrl Pts',(1.31917543061769,1.70460745840382,0.991349264982991));
#9580=CARTESIAN_POINT('Ctrl Pts',(1.34548213209931,1.74894552961493,0.955340251466735));
#9581=CARTESIAN_POINT('Ctrl Pts',(1.36172049302549,1.76817777258318,0.932292094146256));
#9582=CARTESIAN_POINT('Ctrl Pts',(1.39561049050871,1.79370633789704,0.880751161609749));
#9583=CARTESIAN_POINT('Ctrl Pts',(1.4132207435299,1.8,0.85222986989595));
#9584=CARTESIAN_POINT('Ctrl Pts',(1.42894191624432,1.8,0.825000000000001));
#9585=CARTESIAN_POINT('Ctrl Pts',(1.53744468918255,1.55,0.598968970568896));
#9586=CARTESIAN_POINT('Ctrl Pts',(1.53744468918255,1.51855708359447,0.598968970568896));
#9587=CARTESIAN_POINT('Ctrl Pts',(1.53516661651472,1.48505200040818,0.60492118480825));
#9588=CARTESIAN_POINT('Ctrl Pts',(1.52552758004446,1.42347183818157,0.628833667319578));
#9589=CARTESIAN_POINT('Ctrl Pts',(1.51812136280714,1.39539254159618,0.646764802471699));
#9590=CARTESIAN_POINT('Ctrl Pts',(1.50008999307766,1.35105447038507,0.687551581002689));
#9591=CARTESIAN_POINT('Ctrl Pts',(1.48824888379079,1.33182222741682,0.713138492740816));
#9592=CARTESIAN_POINT('Ctrl Pts',(1.46055812562105,1.30629366210296,0.768258557763732));
#9593=CARTESIAN_POINT('Ctrl Pts',(1.44466308895875,1.3,0.797770130104052));
#9594=CARTESIAN_POINT('Ctrl Pts',(1.42894191624432,1.3,0.825000000000001));
#9595=CARTESIAN_POINT('',(0.963525491562421,1.55,0.267616567329818));
#9596=CARTESIAN_POINT('',(0.125,1.55,-0.21650635094611));
#9597=CARTESIAN_POINT('Ctrl Pts',(0.963525491562421,1.55,0.267616567329818));
#9598=CARTESIAN_POINT('Ctrl Pts',(0.963525491562421,1.5815373526696,0.267616567329818));
#9599=CARTESIAN_POINT('Ctrl Pts',(0.961833761492987,1.61508042700263,0.273949373987484));
#9600=CARTESIAN_POINT('Ctrl Pts',(0.954308486908894,1.67663267125761,0.299111603474268));
#9601=CARTESIAN_POINT('Ctrl Pts',(0.948394987258249,1.70465411363682,0.31788699900678));
#9602=CARTESIAN_POINT('Ctrl Pts',(0.933155485613026,1.74889618382539,0.360174810895352));
#9603=CARTESIAN_POINT('Ctrl Pts',(0.92278792026947,1.76811531482682,0.386546956384144));
#9604=CARTESIAN_POINT('Ctrl Pts',(0.897143218189782,1.79367084275751,0.442820664919227));
#9605=CARTESIAN_POINT('Ctrl Pts',(0.881791875377343,1.8,0.472691670144998));
#9606=CARTESIAN_POINT('Ctrl Pts',(0.850258932191534,1.8,0.527308329855003));
#9607=CARTESIAN_POINT('Ctrl Pts',(0.832065554235658,1.79367084275751,0.555538485325664));
#9608=CARTESIAN_POINT('Ctrl Pts',(0.796153444118959,1.76811531482682,0.605884303066698));
#9609=CARTESIAN_POINT('Ctrl Pts',(0.778498278845144,1.74889618382539,0.62804895077401));
#9610=CARTESIAN_POINT('Ctrl Pts',(0.749495710301794,1.70465411363682,0.662390652284073));
#9611=CARTESIAN_POINT('Ctrl Pts',(0.73619249062986,1.67663267125761,0.676899590973058));
#9612=CARTESIAN_POINT('Ctrl Pts',(0.718163997970498,1.61508042700263,0.695997784676728));
#9613=CARTESIAN_POINT('Ctrl Pts',(0.713525491562421,1.5815373526696,0.700629269222037));
#9614=CARTESIAN_POINT('Ctrl Pts',(0.713525491562421,1.5184626473304,0.700629269222037));
#9615=CARTESIAN_POINT('Ctrl Pts',(0.718163997970498,1.48491957299737,0.695997784676728));
#9616=CARTESIAN_POINT('Ctrl Pts',(0.73619249062986,1.42336732874239,0.676899590973058));
#9617=CARTESIAN_POINT('Ctrl Pts',(0.749495710301794,1.39534588636318,0.662390652284073));
#9618=CARTESIAN_POINT('Ctrl Pts',(0.778498278845144,1.35110381617461,0.62804895077401));
#9619=CARTESIAN_POINT('Ctrl Pts',(0.796153444118959,1.33188468517318,0.605884303066698));
#9620=CARTESIAN_POINT('Ctrl Pts',(0.832065554235658,1.30632915724249,0.555538485325664));
#9621=CARTESIAN_POINT('Ctrl Pts',(0.850258932191534,1.3,0.527308329855003));
#9622=CARTESIAN_POINT('Ctrl Pts',(0.881791875377343,1.3,0.472691670144998));
#9623=CARTESIAN_POINT('Ctrl Pts',(0.897143218189782,1.30632915724249,0.442820664919227));
#9624=CARTESIAN_POINT('Ctrl Pts',(0.92278792026947,1.33188468517318,0.386546956384144));
#9625=CARTESIAN_POINT('Ctrl Pts',(0.933155485613026,1.35110381617461,0.360174810895352));
#9626=CARTESIAN_POINT('Ctrl Pts',(0.948394987258249,1.39534588636318,0.31788699900678));
#9627=CARTESIAN_POINT('Ctrl Pts',(0.954308486908894,1.42336732874239,0.299111603474268));
#9628=CARTESIAN_POINT('Ctrl Pts',(0.961833761492987,1.48491957299738,0.273949373987484));
#9629=CARTESIAN_POINT('Ctrl Pts',(0.963525491562421,1.5184626473304,0.267616567329818));
#9630=CARTESIAN_POINT('Ctrl Pts',(0.963525491562421,1.55,0.267616567329818));
#9631=CARTESIAN_POINT('Origin',(0.,1.55,0.));
#9632=CARTESIAN_POINT('',(-0.713525491562421,1.55,-0.700629269222037));
#9633=CARTESIAN_POINT('Ctrl Pts',(-0.713525491562421,1.55,-0.700629269222037));
#9634=CARTESIAN_POINT('Ctrl Pts',(-0.713525491562421,1.5184626473304,-0.700629269222037));
#9635=CARTESIAN_POINT('Ctrl Pts',(-0.718163997970498,1.48491957299737,-0.695997784676728));
#9636=CARTESIAN_POINT('Ctrl Pts',(-0.73619249062986,1.42336732874239,-0.676899590973058));
#9637=CARTESIAN_POINT('Ctrl Pts',(-0.749495710301794,1.39534588636318,-0.662390652284073));
#9638=CARTESIAN_POINT('Ctrl Pts',(-0.778498278845144,1.35110381617461,-0.62804895077401));
#9639=CARTESIAN_POINT('Ctrl Pts',(-0.796153444118959,1.33188468517318,-0.605884303066698));
#9640=CARTESIAN_POINT('Ctrl Pts',(-0.832065554235658,1.30632915724249,-0.555538485325664));
#9641=CARTESIAN_POINT('Ctrl Pts',(-0.850258932191534,1.3,-0.527308329855003));
#9642=CARTESIAN_POINT('Ctrl Pts',(-0.881791875377343,1.3,-0.472691670144998));
#9643=CARTESIAN_POINT('Ctrl Pts',(-0.897143218189782,1.30632915724249,-0.442820664919227));
#9644=CARTESIAN_POINT('Ctrl Pts',(-0.92278792026947,1.33188468517318,-0.386546956384144));
#9645=CARTESIAN_POINT('Ctrl Pts',(-0.933155485613026,1.35110381617461,-0.360174810895352));
#9646=CARTESIAN_POINT('Ctrl Pts',(-0.948394987258249,1.39534588636318,-0.31788699900678));
#9647=CARTESIAN_POINT('Ctrl Pts',(-0.954308486908894,1.42336732874239,-0.299111603474268));
#9648=CARTESIAN_POINT('Ctrl Pts',(-0.961833761492986,1.48491957299737,-0.273949373987484));
#9649=CARTESIAN_POINT('Ctrl Pts',(-0.963525491562421,1.5184626473304,-0.267616567329818));
#9650=CARTESIAN_POINT('Ctrl Pts',(-0.963525491562421,1.5815373526696,-0.267616567329818));
#9651=CARTESIAN_POINT('Ctrl Pts',(-0.961833761492986,1.61508042700263,-0.273949373987484));
#9652=CARTESIAN_POINT('Ctrl Pts',(-0.954308486908894,1.67663267125761,-0.299111603474268));
#9653=CARTESIAN_POINT('Ctrl Pts',(-0.948394987258249,1.70465411363682,-0.31788699900678));
#9654=CARTESIAN_POINT('Ctrl Pts',(-0.933155485613026,1.74889618382539,-0.360174810895352));
#9655=CARTESIAN_POINT('Ctrl Pts',(-0.92278792026947,1.76811531482682,-0.386546956384144));
#9656=CARTESIAN_POINT('Ctrl Pts',(-0.897143218189782,1.79367084275751,-0.442820664919227));
#9657=CARTESIAN_POINT('Ctrl Pts',(-0.881791875377343,1.8,-0.472691670144998));
#9658=CARTESIAN_POINT('Ctrl Pts',(-0.850258932191534,1.8,-0.527308329855003));
#9659=CARTESIAN_POINT('Ctrl Pts',(-0.832065554235658,1.79367084275751,-0.555538485325664));
#9660=CARTESIAN_POINT('Ctrl Pts',(-0.796153444118959,1.76811531482682,-0.605884303066698));
#9661=CARTESIAN_POINT('Ctrl Pts',(-0.778498278845144,1.74889618382539,-0.62804895077401));
#9662=CARTESIAN_POINT('Ctrl Pts',(-0.749495710301794,1.70465411363682,-0.662390652284073));
#9663=CARTESIAN_POINT('Ctrl Pts',(-0.73619249062986,1.67663267125761,-0.676899590973058));
#9664=CARTESIAN_POINT('Ctrl Pts',(-0.718163997970498,1.61508042700263,-0.695997784676728));
#9665=CARTESIAN_POINT('Ctrl Pts',(-0.713525491562421,1.5815373526696,-0.700629269222037));
#9666=CARTESIAN_POINT('Ctrl Pts',(-0.713525491562421,1.55,-0.700629269222037));
#9667=CARTESIAN_POINT('',(-1.28744468918255,1.55,-1.03198167246111));
#9668=CARTESIAN_POINT('',(0.125,1.55,-0.21650635094611));
#9669=CARTESIAN_POINT('',(-1.42894191624432,1.3,-0.825000000000001));
#9670=CARTESIAN_POINT('Ctrl Pts',(-1.42894191624432,1.3,-0.825000000000001));
#9671=CARTESIAN_POINT('Ctrl Pts',(-1.4132207435299,1.3,-0.852229869895949));
#9672=CARTESIAN_POINT('Ctrl Pts',(-1.39561049050871,1.30629366210296,-0.880751161609749));
#9673=CARTESIAN_POINT('Ctrl Pts',(-1.36172049302549,1.33182222741682,-0.932292094146256));
#9674=CARTESIAN_POINT('Ctrl Pts',(-1.34548213209931,1.35105447038507,-0.955340251466735));
#9675=CARTESIAN_POINT('Ctrl Pts',(-1.31917543061769,1.39539254159618,-0.991349264982991));
#9676=CARTESIAN_POINT('Ctrl Pts',(-1.30734972067592,1.42347183818157,-1.00672880483252));
#9677=CARTESIAN_POINT('Ctrl Pts',(-1.29146042158868,1.48505200040818,-1.02703269653942));
#9678=CARTESIAN_POINT('Ctrl Pts',(-1.28744468918255,1.51855708359447,-1.03198167246111));
#9679=CARTESIAN_POINT('Ctrl Pts',(-1.28744468918255,1.55,-1.03198167246111));
#9680=CARTESIAN_POINT('',(-1.42894191624432,1.8,-0.825000000000001));
#9681=CARTESIAN_POINT('Ctrl Pts',(-1.42894191624432,1.8,-0.825000000000001));
#9682=CARTESIAN_POINT('Ctrl Pts',(-1.44466308895875,1.8,-0.797770130104052));
#9683=CARTESIAN_POINT('Ctrl Pts',(-1.46055812562105,1.79370633789704,-0.768258557763732));
#9684=CARTESIAN_POINT('Ctrl Pts',(-1.48824888379079,1.76817777258318,-0.713138492740816));
#9685=CARTESIAN_POINT('Ctrl Pts',(-1.50008999307766,1.74894552961493,-0.687551581002689));
#9686=CARTESIAN_POINT('Ctrl Pts',(-1.51812136280714,1.70460745840382,-0.646764802471699));
#9687=CARTESIAN_POINT('Ctrl Pts',(-1.52552758004446,1.67652816181843,-0.628833667319578));
#9688=CARTESIAN_POINT('Ctrl Pts',(-1.53516661651472,1.61494799959182,-0.60492118480825));
#9689=CARTESIAN_POINT('Ctrl Pts',(-1.53744468918255,1.58144291640553,-0.598968970568896));
#9690=CARTESIAN_POINT('Ctrl Pts',(-1.53744468918255,1.51855708359447,-0.598968970568896));
#9691=CARTESIAN_POINT('Ctrl Pts',(-1.53516661651472,1.48505200040818,-0.60492118480825));
#9692=CARTESIAN_POINT('Ctrl Pts',(-1.52552758004446,1.42347183818157,-0.628833667319578));
#9693=CARTESIAN_POINT('Ctrl Pts',(-1.51812136280714,1.39539254159618,-0.646764802471699));
#9694=CARTESIAN_POINT('Ctrl Pts',(-1.50008999307766,1.35105447038507,-0.687551581002689));
#9695=CARTESIAN_POINT('Ctrl Pts',(-1.48824888379079,1.33182222741682,-0.713138492740816));
#9696=CARTESIAN_POINT('Ctrl Pts',(-1.46055812562105,1.30629366210296,-0.768258557763732));
#9697=CARTESIAN_POINT('Ctrl Pts',(-1.44466308895875,1.3,-0.797770130104052));
#9698=CARTESIAN_POINT('Ctrl Pts',(-1.42894191624432,1.3,-0.825000000000001));
#9699=CARTESIAN_POINT('Ctrl Pts',(-1.28744468918255,1.55,-1.03198167246111));
#9700=CARTESIAN_POINT('Ctrl Pts',(-1.28744468918255,1.58144291640553,-1.03198167246111));
#9701=CARTESIAN_POINT('Ctrl Pts',(-1.29146042158868,1.61494799959182,-1.02703269653942));
#9702=CARTESIAN_POINT('Ctrl Pts',(-1.30734972067592,1.67652816181843,-1.00672880483252));
#9703=CARTESIAN_POINT('Ctrl Pts',(-1.31917543061769,1.70460745840382,-0.991349264982991));
#9704=CARTESIAN_POINT('Ctrl Pts',(-1.34548213209931,1.74894552961493,-0.955340251466734));
#9705=CARTESIAN_POINT('Ctrl Pts',(-1.36172049302549,1.76817777258318,-0.932292094146256));
#9706=CARTESIAN_POINT('Ctrl Pts',(-1.39561049050871,1.79370633789704,-0.880751161609749));
#9707=CARTESIAN_POINT('Ctrl Pts',(-1.4132207435299,1.8,-0.852229869895949));
#9708=CARTESIAN_POINT('Ctrl Pts',(-1.42894191624432,1.8,-0.825000000000001));
#9709=CARTESIAN_POINT('Origin',(0.,1.55,0.));
#9710=CARTESIAN_POINT('',(-1.65,0.85,-2.02066721859313E-16));
#9711=CARTESIAN_POINT('Origin',(0.,0.85,0.));
#9712=CARTESIAN_POINT('',(-1.65,2.25,-2.02066721859313E-16));
#9713=CARTESIAN_POINT('',(-1.65,1.55,-2.02066721859313E-16));
#9714=CARTESIAN_POINT('Origin',(0.,2.25,0.));
#9715=CARTESIAN_POINT('',(-1.42894191624432,1.3,0.825));
#9716=CARTESIAN_POINT('',(-1.42894191624432,1.8,0.825));
#9717=CARTESIAN_POINT('Ctrl Pts',(-1.42894191624432,1.3,0.825));
#9718=CARTESIAN_POINT('Ctrl Pts',(-1.44466308895875,1.3,0.797770130104051));
#9719=CARTESIAN_POINT('Ctrl Pts',(-1.46055812562105,1.30629366210296,0.768258557763731));
#9720=CARTESIAN_POINT('Ctrl Pts',(-1.48824888379079,1.33182222741682,0.713138492740815));
#9721=CARTESIAN_POINT('Ctrl Pts',(-1.50008999307766,1.35105447038507,0.687551581002688));
#9722=CARTESIAN_POINT('Ctrl Pts',(-1.51812136280714,1.39539254159618,0.646764802471698));
#9723=CARTESIAN_POINT('Ctrl Pts',(-1.52552758004446,1.42347183818157,0.628833667319577));
#9724=CARTESIAN_POINT('Ctrl Pts',(-1.53516661651472,1.48505200040818,0.604921184808249));
#9725=CARTESIAN_POINT('Ctrl Pts',(-1.53744468918255,1.51855708359447,0.598968970568895));
#9726=CARTESIAN_POINT('Ctrl Pts',(-1.53744468918255,1.58144291640553,0.598968970568895));
#9727=CARTESIAN_POINT('Ctrl Pts',(-1.53516661651472,1.61494799959182,0.604921184808249));
#9728=CARTESIAN_POINT('Ctrl Pts',(-1.52552758004446,1.67652816181843,0.628833667319577));
#9729=CARTESIAN_POINT('Ctrl Pts',(-1.51812136280714,1.70460745840382,0.646764802471698));
#9730=CARTESIAN_POINT('Ctrl Pts',(-1.50008999307766,1.74894552961493,0.687551581002688));
#9731=CARTESIAN_POINT('Ctrl Pts',(-1.48824888379079,1.76817777258318,0.713138492740815));
#9732=CARTESIAN_POINT('Ctrl Pts',(-1.46055812562105,1.79370633789704,0.768258557763731));
#9733=CARTESIAN_POINT('Ctrl Pts',(-1.44466308895875,1.8,0.797770130104051));
#9734=CARTESIAN_POINT('Ctrl Pts',(-1.42894191624432,1.8,0.825));
#9735=CARTESIAN_POINT('',(-1.28744468918255,1.55,1.03198167246111));
#9736=CARTESIAN_POINT('Ctrl Pts',(-1.42894191624432,1.8,0.825));
#9737=CARTESIAN_POINT('Ctrl Pts',(-1.4132207435299,1.8,0.852229869895948));
#9738=CARTESIAN_POINT('Ctrl Pts',(-1.39561049050871,1.79370633789704,0.880751161609747));
#9739=CARTESIAN_POINT('Ctrl Pts',(-1.36172049302549,1.76817777258318,0.932292094146255));
#9740=CARTESIAN_POINT('Ctrl Pts',(-1.34548213209931,1.74894552961493,0.955340251466733));
#9741=CARTESIAN_POINT('Ctrl Pts',(-1.31917543061769,1.70460745840382,0.991349264982989));
#9742=CARTESIAN_POINT('Ctrl Pts',(-1.30734972067592,1.67652816181843,1.00672880483252));
#9743=CARTESIAN_POINT('Ctrl Pts',(-1.29146042158868,1.61494799959182,1.02703269653942));
#9744=CARTESIAN_POINT('Ctrl Pts',(-1.28744468918255,1.58144291640553,1.03198167246111));
#9745=CARTESIAN_POINT('Ctrl Pts',(-1.28744468918255,1.55,1.03198167246111));
#9746=CARTESIAN_POINT('Ctrl Pts',(-1.28744468918255,1.55,1.03198167246111));
#9747=CARTESIAN_POINT('Ctrl Pts',(-1.28744468918255,1.51855708359447,1.03198167246111));
#9748=CARTESIAN_POINT('Ctrl Pts',(-1.29146042158868,1.48505200040818,1.02703269653942));
#9749=CARTESIAN_POINT('Ctrl Pts',(-1.30734972067592,1.42347183818157,1.00672880483252));
#9750=CARTESIAN_POINT('Ctrl Pts',(-1.31917543061769,1.39539254159618,0.99134926498299));
#9751=CARTESIAN_POINT('Ctrl Pts',(-1.34548213209931,1.35105447038508,0.955340251466733));
#9752=CARTESIAN_POINT('Ctrl Pts',(-1.36172049302549,1.33182222741682,0.932292094146255));
#9753=CARTESIAN_POINT('Ctrl Pts',(-1.39561049050871,1.30629366210296,0.880751161609748));
#9754=CARTESIAN_POINT('Ctrl Pts',(-1.4132207435299,1.3,0.852229869895949));
#9755=CARTESIAN_POINT('Ctrl Pts',(-1.42894191624432,1.3,0.825));
#9756=CARTESIAN_POINT('',(1.42894191624432,1.8,-0.825));
#9757=CARTESIAN_POINT('',(1.42894191624432,1.3,-0.825));
#9758=CARTESIAN_POINT('Ctrl Pts',(1.42894191624432,1.8,-0.825));
#9759=CARTESIAN_POINT('Ctrl Pts',(1.4132207435299,1.8,-0.852229869895949));
#9760=CARTESIAN_POINT('Ctrl Pts',(1.39561049050871,1.79370633789704,-0.880751161609748));
#9761=CARTESIAN_POINT('Ctrl Pts',(1.36172049302549,1.76817777258318,-0.932292094146255));
#9762=CARTESIAN_POINT('Ctrl Pts',(1.34548213209931,1.74894552961493,-0.955340251466734));
#9763=CARTESIAN_POINT('Ctrl Pts',(1.31917543061769,1.70460745840382,-0.99134926498299));
#9764=CARTESIAN_POINT('Ctrl Pts',(1.30734972067592,1.67652816181843,-1.00672880483252));
#9765=CARTESIAN_POINT('Ctrl Pts',(1.29146042158868,1.61494799959182,-1.02703269653942));
#9766=CARTESIAN_POINT('Ctrl Pts',(1.28744468918255,1.58144291640553,-1.03198167246111));
#9767=CARTESIAN_POINT('Ctrl Pts',(1.28744468918255,1.51855708359447,-1.03198167246111));
#9768=CARTESIAN_POINT('Ctrl Pts',(1.29146042158868,1.48505200040818,-1.02703269653942));
#9769=CARTESIAN_POINT('Ctrl Pts',(1.30734972067592,1.42347183818157,-1.00672880483252));
#9770=CARTESIAN_POINT('Ctrl Pts',(1.31917543061769,1.39539254159618,-0.99134926498299));
#9771=CARTESIAN_POINT('Ctrl Pts',(1.34548213209931,1.35105447038507,-0.955340251466734));
#9772=CARTESIAN_POINT('Ctrl Pts',(1.36172049302549,1.33182222741682,-0.932292094146255));
#9773=CARTESIAN_POINT('Ctrl Pts',(1.39561049050871,1.30629366210296,-0.880751161609748));
#9774=CARTESIAN_POINT('Ctrl Pts',(1.4132207435299,1.3,-0.852229869895948));
#9775=CARTESIAN_POINT('Ctrl Pts',(1.42894191624432,1.3,-0.825));
#9776=CARTESIAN_POINT('',(1.53744468918255,1.55,-0.598968970568895));
#9777=CARTESIAN_POINT('Ctrl Pts',(1.42894191624432,1.3,-0.825));
#9778=CARTESIAN_POINT('Ctrl Pts',(1.44466308895875,1.3,-0.797770130104051));
#9779=CARTESIAN_POINT('Ctrl Pts',(1.46055812562105,1.30629366210296,-0.768258557763731));
#9780=CARTESIAN_POINT('Ctrl Pts',(1.48824888379079,1.33182222741682,-0.713138492740815));
#9781=CARTESIAN_POINT('Ctrl Pts',(1.50008999307766,1.35105447038507,-0.687551581002688));
#9782=CARTESIAN_POINT('Ctrl Pts',(1.51812136280714,1.39539254159618,-0.646764802471698));
#9783=CARTESIAN_POINT('Ctrl Pts',(1.52552758004446,1.42347183818157,-0.628833667319577));
#9784=CARTESIAN_POINT('Ctrl Pts',(1.53516661651472,1.48505200040818,-0.604921184808249));
#9785=CARTESIAN_POINT('Ctrl Pts',(1.53744468918255,1.51855708359447,-0.598968970568895));
#9786=CARTESIAN_POINT('Ctrl Pts',(1.53744468918255,1.55,-0.598968970568895));
#9787=CARTESIAN_POINT('Ctrl Pts',(1.53744468918255,1.55,-0.598968970568895));
#9788=CARTESIAN_POINT('Ctrl Pts',(1.53744468918255,1.58144291640553,-0.598968970568895));
#9789=CARTESIAN_POINT('Ctrl Pts',(1.53516661651472,1.61494799959182,-0.604921184808249));
#9790=CARTESIAN_POINT('Ctrl Pts',(1.52552758004446,1.67652816181843,-0.628833667319577));
#9791=CARTESIAN_POINT('Ctrl Pts',(1.51812136280714,1.70460745840382,-0.646764802471698));
#9792=CARTESIAN_POINT('Ctrl Pts',(1.50008999307766,1.74894552961493,-0.687551581002688));
#9793=CARTESIAN_POINT('Ctrl Pts',(1.48824888379079,1.76817777258318,-0.713138492740815));
#9794=CARTESIAN_POINT('Ctrl Pts',(1.46055812562105,1.79370633789704,-0.768258557763731));
#9795=CARTESIAN_POINT('Ctrl Pts',(1.44466308895875,1.8,-0.797770130104051));
#9796=CARTESIAN_POINT('Ctrl Pts',(1.42894191624432,1.8,-0.825));
#9797=CARTESIAN_POINT('',(0.,1.3,-1.65));
#9798=CARTESIAN_POINT('',(0.,1.8,-1.65));
#9799=CARTESIAN_POINT('Ctrl Pts',(1.38777878078145E-17,1.3,-1.65));
#9800=CARTESIAN_POINT('Ctrl Pts',(0.0314423454288489,1.3,-1.65));
#9801=CARTESIAN_POINT('Ctrl Pts',(0.0649476351123396,1.30629366210296,-1.64900971937348));
#9802=CARTESIAN_POINT('Ctrl Pts',(0.126528390765307,1.33182222741682,-1.64543058688707));
#9803=CARTESIAN_POINT('Ctrl Pts',(0.154607860978348,1.35105447038507,-1.64289183246942));
#9804=CARTESIAN_POINT('Ctrl Pts',(0.198945932189457,1.39539254159618,-1.63811406745469));
#9805=CARTESIAN_POINT('Ctrl Pts',(0.218177859368546,1.42347183818157,-1.63556247215209));
#9806=CARTESIAN_POINT('Ctrl Pts',(0.243706194926033,1.48505200040818,-1.63195388134767));
#9807=CARTESIAN_POINT('Ctrl Pts',(0.25,1.51855708359447,-1.63095064303001));
#9808=CARTESIAN_POINT('Ctrl Pts',(0.25,1.58144291640553,-1.63095064303001));
#9809=CARTESIAN_POINT('Ctrl Pts',(0.243706194926033,1.61494799959182,-1.63195388134767));
#9810=CARTESIAN_POINT('Ctrl Pts',(0.218177859368546,1.67652816181843,-1.63556247215209));
#9811=CARTESIAN_POINT('Ctrl Pts',(0.198945932189457,1.70460745840382,-1.63811406745469));
#9812=CARTESIAN_POINT('Ctrl Pts',(0.154607860978349,1.74894552961493,-1.64289183246942));
#9813=CARTESIAN_POINT('Ctrl Pts',(0.126528390765307,1.76817777258318,-1.64543058688707));
#9814=CARTESIAN_POINT('Ctrl Pts',(0.0649476351123398,1.79370633789704,-1.64900971937348));
#9815=CARTESIAN_POINT('Ctrl Pts',(0.031442345428849,1.8,-1.65));
#9816=CARTESIAN_POINT('Ctrl Pts',(7.63278329429795E-17,1.8,-1.65));
#9817=CARTESIAN_POINT('',(-0.25,1.55,-1.63095064303001));
#9818=CARTESIAN_POINT('Ctrl Pts',(9.0205620750794E-17,1.8,-1.65));
#9819=CARTESIAN_POINT('Ctrl Pts',(-0.0314423454288488,1.8,-1.65));
#9820=CARTESIAN_POINT('Ctrl Pts',(-0.0649476351123396,1.79370633789704,
-1.64900971937348));
#9821=CARTESIAN_POINT('Ctrl Pts',(-0.126528390765307,1.76817777258318,-1.64543058688707));
#9822=CARTESIAN_POINT('Ctrl Pts',(-0.154607860978348,1.74894552961493,-1.64289183246942));
#9823=CARTESIAN_POINT('Ctrl Pts',(-0.198945932189456,1.70460745840382,-1.63811406745469));
#9824=CARTESIAN_POINT('Ctrl Pts',(-0.218177859368546,1.67652816181843,-1.63556247215209));
#9825=CARTESIAN_POINT('Ctrl Pts',(-0.243706194926033,1.61494799959182,-1.63195388134767));
#9826=CARTESIAN_POINT('Ctrl Pts',(-0.25,1.58144291640553,-1.63095064303001));
#9827=CARTESIAN_POINT('Ctrl Pts',(-0.25,1.55,-1.63095064303001));
#9828=CARTESIAN_POINT('Ctrl Pts',(-0.25,1.55,-1.63095064303001));
#9829=CARTESIAN_POINT('Ctrl Pts',(-0.25,1.51855708359447,-1.63095064303001));
#9830=CARTESIAN_POINT('Ctrl Pts',(-0.243706194926033,1.48505200040818,-1.63195388134767));
#9831=CARTESIAN_POINT('Ctrl Pts',(-0.218177859368546,1.42347183818157,-1.63556247215209));
#9832=CARTESIAN_POINT('Ctrl Pts',(-0.198945932189457,1.39539254159618,-1.63811406745469));
#9833=CARTESIAN_POINT('Ctrl Pts',(-0.154607860978349,1.35105447038507,-1.64289183246942));
#9834=CARTESIAN_POINT('Ctrl Pts',(-0.126528390765307,1.33182222741682,-1.64543058688707));
#9835=CARTESIAN_POINT('Ctrl Pts',(-0.0649476351123398,1.30629366210296,
-1.64900971937348));
#9836=CARTESIAN_POINT('Ctrl Pts',(-0.031442345428849,1.3,-1.65));
#9837=CARTESIAN_POINT('Ctrl Pts',(-4.85722573273506E-17,1.3,-1.65));
#9838=CARTESIAN_POINT('',(0.,1.8,1.65));
#9839=CARTESIAN_POINT('',(0.,1.3,1.65));
#9840=CARTESIAN_POINT('Ctrl Pts',(8.32667268468867E-17,1.8,1.65));
#9841=CARTESIAN_POINT('Ctrl Pts',(0.031442345428849,1.8,1.65));
#9842=CARTESIAN_POINT('Ctrl Pts',(0.0649476351123398,1.79370633789704,1.64900971937348));
#9843=CARTESIAN_POINT('Ctrl Pts',(0.126528390765307,1.76817777258318,1.64543058688707));
#9844=CARTESIAN_POINT('Ctrl Pts',(0.154607860978349,1.74894552961493,1.64289183246942));
#9845=CARTESIAN_POINT('Ctrl Pts',(0.198945932189457,1.70460745840382,1.63811406745469));
#9846=CARTESIAN_POINT('Ctrl Pts',(0.218177859368546,1.67652816181843,1.63556247215209));
#9847=CARTESIAN_POINT('Ctrl Pts',(0.243706194926033,1.61494799959182,1.63195388134767));
#9848=CARTESIAN_POINT('Ctrl Pts',(0.25,1.58144291640553,1.63095064303001));
#9849=CARTESIAN_POINT('Ctrl Pts',(0.25,1.51855708359447,1.63095064303001));
#9850=CARTESIAN_POINT('Ctrl Pts',(0.243706194926033,1.48505200040818,1.63195388134767));
#9851=CARTESIAN_POINT('Ctrl Pts',(0.218177859368546,1.42347183818157,1.63556247215209));
#9852=CARTESIAN_POINT('Ctrl Pts',(0.198945932189457,1.39539254159618,1.63811406745469));
#9853=CARTESIAN_POINT('Ctrl Pts',(0.154607860978348,1.35105447038507,1.64289183246942));
#9854=CARTESIAN_POINT('Ctrl Pts',(0.126528390765307,1.33182222741682,1.64543058688707));
#9855=CARTESIAN_POINT('Ctrl Pts',(0.0649476351123397,1.30629366210296,1.64900971937348));
#9856=CARTESIAN_POINT('Ctrl Pts',(0.0314423454288488,1.3,1.65));
#9857=CARTESIAN_POINT('Ctrl Pts',(-1.38777878078145E-17,1.3,1.65));
#9858=CARTESIAN_POINT('',(-0.25,1.55,1.63095064303001));
#9859=CARTESIAN_POINT('Ctrl Pts',(-5.55111512312578E-17,1.3,1.65));
#9860=CARTESIAN_POINT('Ctrl Pts',(-0.031442345428849,1.3,1.65));
#9861=CARTESIAN_POINT('Ctrl Pts',(-0.0649476351123398,1.30629366210296,
1.64900971937348));
#9862=CARTESIAN_POINT('Ctrl Pts',(-0.126528390765307,1.33182222741682,1.64543058688707));
#9863=CARTESIAN_POINT('Ctrl Pts',(-0.154607860978349,1.35105447038507,1.64289183246942));
#9864=CARTESIAN_POINT('Ctrl Pts',(-0.198945932189457,1.39539254159618,1.63811406745469));
#9865=CARTESIAN_POINT('Ctrl Pts',(-0.218177859368546,1.42347183818157,1.63556247215209));
#9866=CARTESIAN_POINT('Ctrl Pts',(-0.243706194926033,1.48505200040818,1.63195388134767));
#9867=CARTESIAN_POINT('Ctrl Pts',(-0.25,1.51855708359447,1.63095064303001));
#9868=CARTESIAN_POINT('Ctrl Pts',(-0.25,1.55,1.63095064303001));
#9869=CARTESIAN_POINT('Ctrl Pts',(-0.25,1.55,1.63095064303001));
#9870=CARTESIAN_POINT('Ctrl Pts',(-0.25,1.58144291640553,1.63095064303001));
#9871=CARTESIAN_POINT('Ctrl Pts',(-0.243706194926033,1.61494799959182,1.63195388134767));
#9872=CARTESIAN_POINT('Ctrl Pts',(-0.218177859368546,1.67652816181843,1.63556247215209));
#9873=CARTESIAN_POINT('Ctrl Pts',(-0.198945932189456,1.70460745840382,1.63811406745469));
#9874=CARTESIAN_POINT('Ctrl Pts',(-0.154607860978348,1.74894552961493,1.64289183246942));
#9875=CARTESIAN_POINT('Ctrl Pts',(-0.126528390765307,1.76817777258318,1.64543058688707));
#9876=CARTESIAN_POINT('Ctrl Pts',(-0.0649476351123396,1.79370633789704,
1.64900971937348));
#9877=CARTESIAN_POINT('Ctrl Pts',(-0.0314423454288488,1.8,1.65));
#9878=CARTESIAN_POINT('Ctrl Pts',(7.63278329429795E-17,1.8,1.65));
#9879=CARTESIAN_POINT('Origin',(0.,1.55,0.));
#9880=CARTESIAN_POINT('',(-0.713525491562421,1.55,0.700629269222037));
#9881=CARTESIAN_POINT('',(0.125,1.55,0.21650635094611));
#9882=CARTESIAN_POINT('Ctrl Pts',(-0.713525491562421,1.55,0.700629269222037));
#9883=CARTESIAN_POINT('Ctrl Pts',(-0.713525491562421,1.5815373526696,0.700629269222037));
#9884=CARTESIAN_POINT('Ctrl Pts',(-0.718163997970498,1.61508042700263,0.695997784676727));
#9885=CARTESIAN_POINT('Ctrl Pts',(-0.73619249062986,1.67663267125761,0.676899590973058));
#9886=CARTESIAN_POINT('Ctrl Pts',(-0.749495710301795,1.70465411363682,0.662390652284073));
#9887=CARTESIAN_POINT('Ctrl Pts',(-0.778498278845144,1.74889618382539,0.628048950774009));
#9888=CARTESIAN_POINT('Ctrl Pts',(-0.796153444118959,1.76811531482682,0.605884303066698));
#9889=CARTESIAN_POINT('Ctrl Pts',(-0.832065554235658,1.79367084275751,0.555538485325663));
#9890=CARTESIAN_POINT('Ctrl Pts',(-0.850258932191534,1.8,0.527308329855002));
#9891=CARTESIAN_POINT('Ctrl Pts',(-0.881791875377343,1.8,0.472691670144998));
#9892=CARTESIAN_POINT('Ctrl Pts',(-0.897143218189782,1.79367084275751,0.442820664919227));
#9893=CARTESIAN_POINT('Ctrl Pts',(-0.92278792026947,1.76811531482682,0.386546956384144));
#9894=CARTESIAN_POINT('Ctrl Pts',(-0.933155485613026,1.74889618382539,0.360174810895352));
#9895=CARTESIAN_POINT('Ctrl Pts',(-0.948394987258249,1.70465411363682,0.31788699900678));
#9896=CARTESIAN_POINT('Ctrl Pts',(-0.954308486908894,1.67663267125761,0.299111603474267));
#9897=CARTESIAN_POINT('Ctrl Pts',(-0.961833761492987,1.61508042700263,0.273949373987484));
#9898=CARTESIAN_POINT('Ctrl Pts',(-0.963525491562421,1.5815373526696,0.267616567329817));
#9899=CARTESIAN_POINT('Ctrl Pts',(-0.963525491562421,1.5184626473304,0.267616567329817));
#9900=CARTESIAN_POINT('Ctrl Pts',(-0.961833761492987,1.48491957299737,0.273949373987484));
#9901=CARTESIAN_POINT('Ctrl Pts',(-0.954308486908894,1.42336732874239,0.299111603474267));
#9902=CARTESIAN_POINT('Ctrl Pts',(-0.948394987258249,1.39534588636318,0.31788699900678));
#9903=CARTESIAN_POINT('Ctrl Pts',(-0.933155485613026,1.35110381617461,0.360174810895352));
#9904=CARTESIAN_POINT('Ctrl Pts',(-0.92278792026947,1.33188468517318,0.386546956384144));
#9905=CARTESIAN_POINT('Ctrl Pts',(-0.897143218189782,1.30632915724249,0.442820664919227));
#9906=CARTESIAN_POINT('Ctrl Pts',(-0.881791875377343,1.3,0.472691670144998));
#9907=CARTESIAN_POINT('Ctrl Pts',(-0.850258932191534,1.3,0.527308329855002));
#9908=CARTESIAN_POINT('Ctrl Pts',(-0.832065554235658,1.30632915724249,0.555538485325663));
#9909=CARTESIAN_POINT('Ctrl Pts',(-0.796153444118959,1.33188468517318,0.605884303066698));
#9910=CARTESIAN_POINT('Ctrl Pts',(-0.778498278845144,1.35110381617461,0.628048950774009));
#9911=CARTESIAN_POINT('Ctrl Pts',(-0.749495710301795,1.39534588636318,0.662390652284073));
#9912=CARTESIAN_POINT('Ctrl Pts',(-0.73619249062986,1.42336732874239,0.676899590973058));
#9913=CARTESIAN_POINT('Ctrl Pts',(-0.718163997970498,1.48491957299737,0.695997784676727));
#9914=CARTESIAN_POINT('Ctrl Pts',(-0.713525491562421,1.5184626473304,0.700629269222037));
#9915=CARTESIAN_POINT('Ctrl Pts',(-0.713525491562421,1.55,0.700629269222037));
#9916=CARTESIAN_POINT('Origin',(0.,1.55,0.));
#9917=CARTESIAN_POINT('',(0.963525491562421,1.55,-0.267616567329817));
#9918=CARTESIAN_POINT('Ctrl Pts',(0.963525491562421,1.55,-0.267616567329817));
#9919=CARTESIAN_POINT('Ctrl Pts',(0.963525491562421,1.5184626473304,-0.267616567329817));
#9920=CARTESIAN_POINT('Ctrl Pts',(0.961833761492987,1.48491957299737,-0.273949373987484));
#9921=CARTESIAN_POINT('Ctrl Pts',(0.954308486908894,1.42336732874239,-0.299111603474267));
#9922=CARTESIAN_POINT('Ctrl Pts',(0.948394987258249,1.39534588636318,-0.31788699900678));
#9923=CARTESIAN_POINT('Ctrl Pts',(0.933155485613026,1.35110381617461,-0.360174810895352));
#9924=CARTESIAN_POINT('Ctrl Pts',(0.92278792026947,1.33188468517318,-0.386546956384144));
#9925=CARTESIAN_POINT('Ctrl Pts',(0.897143218189782,1.30632915724249,-0.442820664919227));
#9926=CARTESIAN_POINT('Ctrl Pts',(0.881791875377343,1.3,-0.472691670144998));
#9927=CARTESIAN_POINT('Ctrl Pts',(0.850258932191534,1.3,-0.527308329855002));
#9928=CARTESIAN_POINT('Ctrl Pts',(0.832065554235658,1.30632915724249,-0.555538485325663));
#9929=CARTESIAN_POINT('Ctrl Pts',(0.796153444118959,1.33188468517318,-0.605884303066698));
#9930=CARTESIAN_POINT('Ctrl Pts',(0.778498278845144,1.35110381617461,-0.628048950774009));
#9931=CARTESIAN_POINT('Ctrl Pts',(0.749495710301795,1.39534588636318,-0.662390652284073));
#9932=CARTESIAN_POINT('Ctrl Pts',(0.73619249062986,1.42336732874239,-0.676899590973058));
#9933=CARTESIAN_POINT('Ctrl Pts',(0.718163997970498,1.48491957299737,-0.695997784676727));
#9934=CARTESIAN_POINT('Ctrl Pts',(0.713525491562421,1.5184626473304,-0.700629269222037));
#9935=CARTESIAN_POINT('Ctrl Pts',(0.713525491562421,1.5815373526696,-0.700629269222037));
#9936=CARTESIAN_POINT('Ctrl Pts',(0.718163997970498,1.61508042700263,-0.695997784676727));
#9937=CARTESIAN_POINT('Ctrl Pts',(0.73619249062986,1.67663267125761,-0.676899590973058));
#9938=CARTESIAN_POINT('Ctrl Pts',(0.749495710301795,1.70465411363682,-0.662390652284073));
#9939=CARTESIAN_POINT('Ctrl Pts',(0.778498278845144,1.74889618382539,-0.628048950774009));
#9940=CARTESIAN_POINT('Ctrl Pts',(0.796153444118959,1.76811531482682,-0.605884303066698));
#9941=CARTESIAN_POINT('Ctrl Pts',(0.832065554235658,1.79367084275751,-0.555538485325663));
#9942=CARTESIAN_POINT('Ctrl Pts',(0.850258932191534,1.8,-0.527308329855002));
#9943=CARTESIAN_POINT('Ctrl Pts',(0.881791875377343,1.8,-0.472691670144998));
#9944=CARTESIAN_POINT('Ctrl Pts',(0.897143218189782,1.79367084275751,-0.442820664919227));
#9945=CARTESIAN_POINT('Ctrl Pts',(0.92278792026947,1.76811531482682,-0.386546956384144));
#9946=CARTESIAN_POINT('Ctrl Pts',(0.933155485613026,1.74889618382539,-0.360174810895352));
#9947=CARTESIAN_POINT('Ctrl Pts',(0.948394987258249,1.70465411363682,-0.31788699900678));
#9948=CARTESIAN_POINT('Ctrl Pts',(0.954308486908894,1.67663267125761,-0.299111603474267));
#9949=CARTESIAN_POINT('Ctrl Pts',(0.961833761492987,1.61508042700263,-0.273949373987484));
#9950=CARTESIAN_POINT('Ctrl Pts',(0.963525491562421,1.5815373526696,-0.267616567329817));
#9951=CARTESIAN_POINT('Ctrl Pts',(0.963525491562421,1.55,-0.267616567329817));
#9952=CARTESIAN_POINT('',(0.125,1.55,0.21650635094611));
#9953=CARTESIAN_POINT('Origin',(0.,1.55,0.));
#9954=CARTESIAN_POINT('',(-0.25,1.55,-0.968245836551854));
#9955=CARTESIAN_POINT('',(-0.25,1.55,0.));
#9956=CARTESIAN_POINT('Ctrl Pts',(-0.25,1.55,-0.968245836551854));
#9957=CARTESIAN_POINT('Ctrl Pts',(-0.25,1.5815373526696,-0.968245836551854));
#9958=CARTESIAN_POINT('Ctrl Pts',(-0.243669763522489,1.61508042700263,-0.969947158664211));
#9959=CARTESIAN_POINT('Ctrl Pts',(-0.218115996279034,1.67663267125761,-0.976011194447325));
#9960=CARTESIAN_POINT('Ctrl Pts',(-0.198899276956455,1.70465411363682,-0.980277651290853));
#9961=CARTESIAN_POINT('Ctrl Pts',(-0.154657206767882,1.74889618382539,-0.988223761669361));
#9962=CARTESIAN_POINT('Ctrl Pts',(-0.126634476150511,1.76811531482682,-0.992431259450842));
#9963=CARTESIAN_POINT('Ctrl Pts',(-0.0650776639541238,1.79367084275751,
-0.99835915024489));
#9964=CARTESIAN_POINT('Ctrl Pts',(-0.0315329431858092,1.8,-1.));
#9965=CARTESIAN_POINT('Ctrl Pts',(0.0315329431858092,1.8,-1.));
#9966=CARTESIAN_POINT('Ctrl Pts',(0.0650776639541238,1.79367084275751,-0.99835915024489));
#9967=CARTESIAN_POINT('Ctrl Pts',(0.126634476150511,1.76811531482682,-0.992431259450842));
#9968=CARTESIAN_POINT('Ctrl Pts',(0.154657206767882,1.74889618382539,-0.988223761669361));
#9969=CARTESIAN_POINT('Ctrl Pts',(0.198899276956455,1.70465411363682,-0.980277651290853));
#9970=CARTESIAN_POINT('Ctrl Pts',(0.218115996279034,1.67663267125761,-0.976011194447325));
#9971=CARTESIAN_POINT('Ctrl Pts',(0.243669763522488,1.61508042700263,-0.969947158664211));
#9972=CARTESIAN_POINT('Ctrl Pts',(0.25,1.5815373526696,-0.968245836551854));
#9973=CARTESIAN_POINT('Ctrl Pts',(0.25,1.5184626473304,-0.968245836551854));
#9974=CARTESIAN_POINT('Ctrl Pts',(0.243669763522488,1.48491957299737,-0.969947158664211));
#9975=CARTESIAN_POINT('Ctrl Pts',(0.218115996279034,1.42336732874239,-0.976011194447325));
#9976=CARTESIAN_POINT('Ctrl Pts',(0.198899276956455,1.39534588636318,-0.980277651290853));
#9977=CARTESIAN_POINT('Ctrl Pts',(0.154657206767882,1.35110381617461,-0.988223761669361));
#9978=CARTESIAN_POINT('Ctrl Pts',(0.126634476150511,1.33188468517318,-0.992431259450842));
#9979=CARTESIAN_POINT('Ctrl Pts',(0.0650776639541239,1.30632915724249,-0.99835915024489));
#9980=CARTESIAN_POINT('Ctrl Pts',(0.0315329431858092,1.3,-1.));
#9981=CARTESIAN_POINT('Ctrl Pts',(-0.0315329431858092,1.3,-1.));
#9982=CARTESIAN_POINT('Ctrl Pts',(-0.0650776639541239,1.30632915724249,
-0.99835915024489));
#9983=CARTESIAN_POINT('Ctrl Pts',(-0.126634476150511,1.33188468517318,-0.992431259450842));
#9984=CARTESIAN_POINT('Ctrl Pts',(-0.154657206767882,1.35110381617461,-0.988223761669361));
#9985=CARTESIAN_POINT('Ctrl Pts',(-0.198899276956455,1.39534588636318,-0.980277651290853));
#9986=CARTESIAN_POINT('Ctrl Pts',(-0.218115996279034,1.42336732874239,-0.976011194447325));
#9987=CARTESIAN_POINT('Ctrl Pts',(-0.243669763522489,1.48491957299737,-0.969947158664211));
#9988=CARTESIAN_POINT('Ctrl Pts',(-0.25,1.5184626473304,-0.968245836551854));
#9989=CARTESIAN_POINT('Ctrl Pts',(-0.25,1.55,-0.968245836551854));
#9990=CARTESIAN_POINT('Origin',(0.,1.55,0.));
#9991=CARTESIAN_POINT('',(-0.25,1.55,0.968245836551854));
#9992=CARTESIAN_POINT('Ctrl Pts',(-0.25,1.55,0.968245836551854));
#9993=CARTESIAN_POINT('Ctrl Pts',(-0.25,1.5184626473304,0.968245836551854));
#9994=CARTESIAN_POINT('Ctrl Pts',(-0.243669763522489,1.48491957299737,0.969947158664211));
#9995=CARTESIAN_POINT('Ctrl Pts',(-0.218115996279034,1.42336732874239,0.976011194447325));
#9996=CARTESIAN_POINT('Ctrl Pts',(-0.198899276956455,1.39534588636318,0.980277651290853));
#9997=CARTESIAN_POINT('Ctrl Pts',(-0.154657206767882,1.35110381617461,0.988223761669361));
#9998=CARTESIAN_POINT('Ctrl Pts',(-0.126634476150511,1.33188468517318,0.992431259450842));
#9999=CARTESIAN_POINT('Ctrl Pts',(-0.065077663954124,1.30632915724249,0.99835915024489));
#10000=CARTESIAN_POINT('Ctrl Pts',(-0.0315329431858092,1.3,1.));
#10001=CARTESIAN_POINT('Ctrl Pts',(0.0315329431858092,1.3,1.));
#10002=CARTESIAN_POINT('Ctrl Pts',(0.065077663954124,1.30632915724249,0.99835915024489));
#10003=CARTESIAN_POINT('Ctrl Pts',(0.126634476150511,1.33188468517318,0.992431259450842));
#10004=CARTESIAN_POINT('Ctrl Pts',(0.154657206767882,1.35110381617461,0.988223761669361));
#10005=CARTESIAN_POINT('Ctrl Pts',(0.198899276956455,1.39534588636318,0.980277651290853));
#10006=CARTESIAN_POINT('Ctrl Pts',(0.218115996279034,1.42336732874239,0.976011194447325));
#10007=CARTESIAN_POINT('Ctrl Pts',(0.243669763522488,1.48491957299737,0.969947158664211));
#10008=CARTESIAN_POINT('Ctrl Pts',(0.25,1.5184626473304,0.968245836551854));
#10009=CARTESIAN_POINT('Ctrl Pts',(0.25,1.5815373526696,0.968245836551854));
#10010=CARTESIAN_POINT('Ctrl Pts',(0.243669763522488,1.61508042700263,0.969947158664211));
#10011=CARTESIAN_POINT('Ctrl Pts',(0.218115996279034,1.67663267125761,0.976011194447325));
#10012=CARTESIAN_POINT('Ctrl Pts',(0.198899276956455,1.70465411363682,0.980277651290853));
#10013=CARTESIAN_POINT('Ctrl Pts',(0.154657206767882,1.74889618382539,0.988223761669361));
#10014=CARTESIAN_POINT('Ctrl Pts',(0.126634476150511,1.76811531482682,0.992431259450842));
#10015=CARTESIAN_POINT('Ctrl Pts',(0.0650776639541239,1.79367084275751,
0.99835915024489));
#10016=CARTESIAN_POINT('Ctrl Pts',(0.0315329431858092,1.8,1.));
#10017=CARTESIAN_POINT('Ctrl Pts',(-0.0315329431858092,1.8,1.));
#10018=CARTESIAN_POINT('Ctrl Pts',(-0.0650776639541239,1.79367084275751,
0.99835915024489));
#10019=CARTESIAN_POINT('Ctrl Pts',(-0.126634476150511,1.76811531482682,
0.992431259450842));
#10020=CARTESIAN_POINT('Ctrl Pts',(-0.154657206767882,1.74889618382539,
0.988223761669361));
#10021=CARTESIAN_POINT('Ctrl Pts',(-0.198899276956455,1.70465411363682,
0.980277651290853));
#10022=CARTESIAN_POINT('Ctrl Pts',(-0.218115996279034,1.67663267125761,
0.976011194447325));
#10023=CARTESIAN_POINT('Ctrl Pts',(-0.243669763522489,1.61508042700263,
0.969947158664211));
#10024=CARTESIAN_POINT('Ctrl Pts',(-0.25,1.5815373526696,0.968245836551854));
#10025=CARTESIAN_POINT('Ctrl Pts',(-0.25,1.55,0.968245836551854));
#10026=CARTESIAN_POINT('',(-0.25,1.55,0.));
#10027=CARTESIAN_POINT('Origin',(1.65,2.25,0.));
#10028=CARTESIAN_POINT('',(-1.,2.25,-1.22464679914735E-16));
#10029=CARTESIAN_POINT('Origin',(0.,2.25,0.));
#10030=CARTESIAN_POINT('Origin',(1.75,0.85,0.));
#10031=CARTESIAN_POINT('',(-1.75,0.85,-2.14313189850787E-16));
#10032=CARTESIAN_POINT('Origin',(0.,0.85,0.));
#10033=CARTESIAN_POINT('Origin',(0.,0.,0.));
#10034=CARTESIAN_POINT('',(-1.75,-0.85,-2.14313189850787E-16));
#10035=CARTESIAN_POINT('Origin',(0.,-0.85,0.));
#10036=CARTESIAN_POINT('',(-1.75,0.,-2.14313189850787E-16));
#10037=CARTESIAN_POINT('Origin',(1.,-0.85,0.));
#10038=CARTESIAN_POINT('',(-1.,-0.85,-1.22464679914735E-16));
#10039=CARTESIAN_POINT('Origin',(0.,-0.85,0.));
#10040=CARTESIAN_POINT('Origin',(0.,0.7,0.));
#10041=CARTESIAN_POINT('',(-1.,0.7,-1.22464679914735E-16));
#11714=UNCERTAINTY_MEASURE_WITH_UNIT(LENGTH_MEASURE(0.001),#11765,
'DISTANCE_ACCURACY_VALUE',
'Maximum model space distance between geometric entities at asserted c
onnectivities');
#11732=UNCERTAINTY_MEASURE_WITH_UNIT(LENGTH_MEASURE(0.001),#11765,
'DISTANCE_ACCURACY_VALUE',
'Maximum model space distance between geometric entities at asserted c
onnectivities');
#11746=(
GEOMETRIC_REPRESENTATION_CONTEXT(3)
GLOBAL_UNCERTAINTY_ASSIGNED_CONTEXT((#11714))
GLOBAL_UNIT_ASSIGNED_CONTEXT((#11765,#11767,#11768))
REPRESENTATION_CONTEXT('','3D')
);
#11764=(
GEOMETRIC_REPRESENTATION_CONTEXT(3)
GLOBAL_UNCERTAINTY_ASSIGNED_CONTEXT((#11732))
GLOBAL_UNIT_ASSIGNED_CONTEXT((#11765,#11767,#11768))
REPRESENTATION_CONTEXT('','3D')
);
#11765=(
LENGTH_UNIT()
NAMED_UNIT(*)
SI_UNIT(.CENTI.,.METRE.)
);
#11767=(
NAMED_UNIT(*)
PLANE_ANGLE_UNIT()
SI_UNIT($,.RADIAN.)
);
#11768=(
NAMED_UNIT(*)
SI_UNIT($,.STERADIAN.)
SOLID_ANGLE_UNIT()
);
#11782=SHAPE_DEFINITION_REPRESENTATION(#11813,#11891);
#11813=PRODUCT_DEFINITION_SHAPE('',$,#11923);
#11891=SHAPE_REPRESENTATION('',(#6618),#11746);
#11909=PRODUCT_DEFINITION_CONTEXT('part definition',#12004,'design');
#11923=PRODUCT_DEFINITION('Insert bearing','Insert bearing',#11954,#11909);
#11954=PRODUCT_DEFINITION_FORMATION('',$,#12019);
#12004=APPLICATION_CONTEXT(
'Core Data for Automotive Mechanical Design Process');
#12005=PRODUCT_CONTEXT('part definition',#12004,'mechanical');
#12019=PRODUCT('Insert bearing','Insert bearing','Insert bearing',(#12005));
#12093=COLOUR_RGB('Grey',0.48,0.52,0.57);
#12094=FILL_AREA_STYLE_COLOUR('',#12093);
#12095=FILL_AREA_STYLE('',(#12094));
#12096=SURFACE_STYLE_FILL_AREA(#12095);
#12097=SURFACE_SIDE_STYLE('',(#12096));
#12098=SURFACE_STYLE_USAGE(.BOTH.,#12097);
#12099=PRESENTATION_STYLE_ASSIGNMENT((#12098));
ENDSEC;
END-ISO-10303-21;
